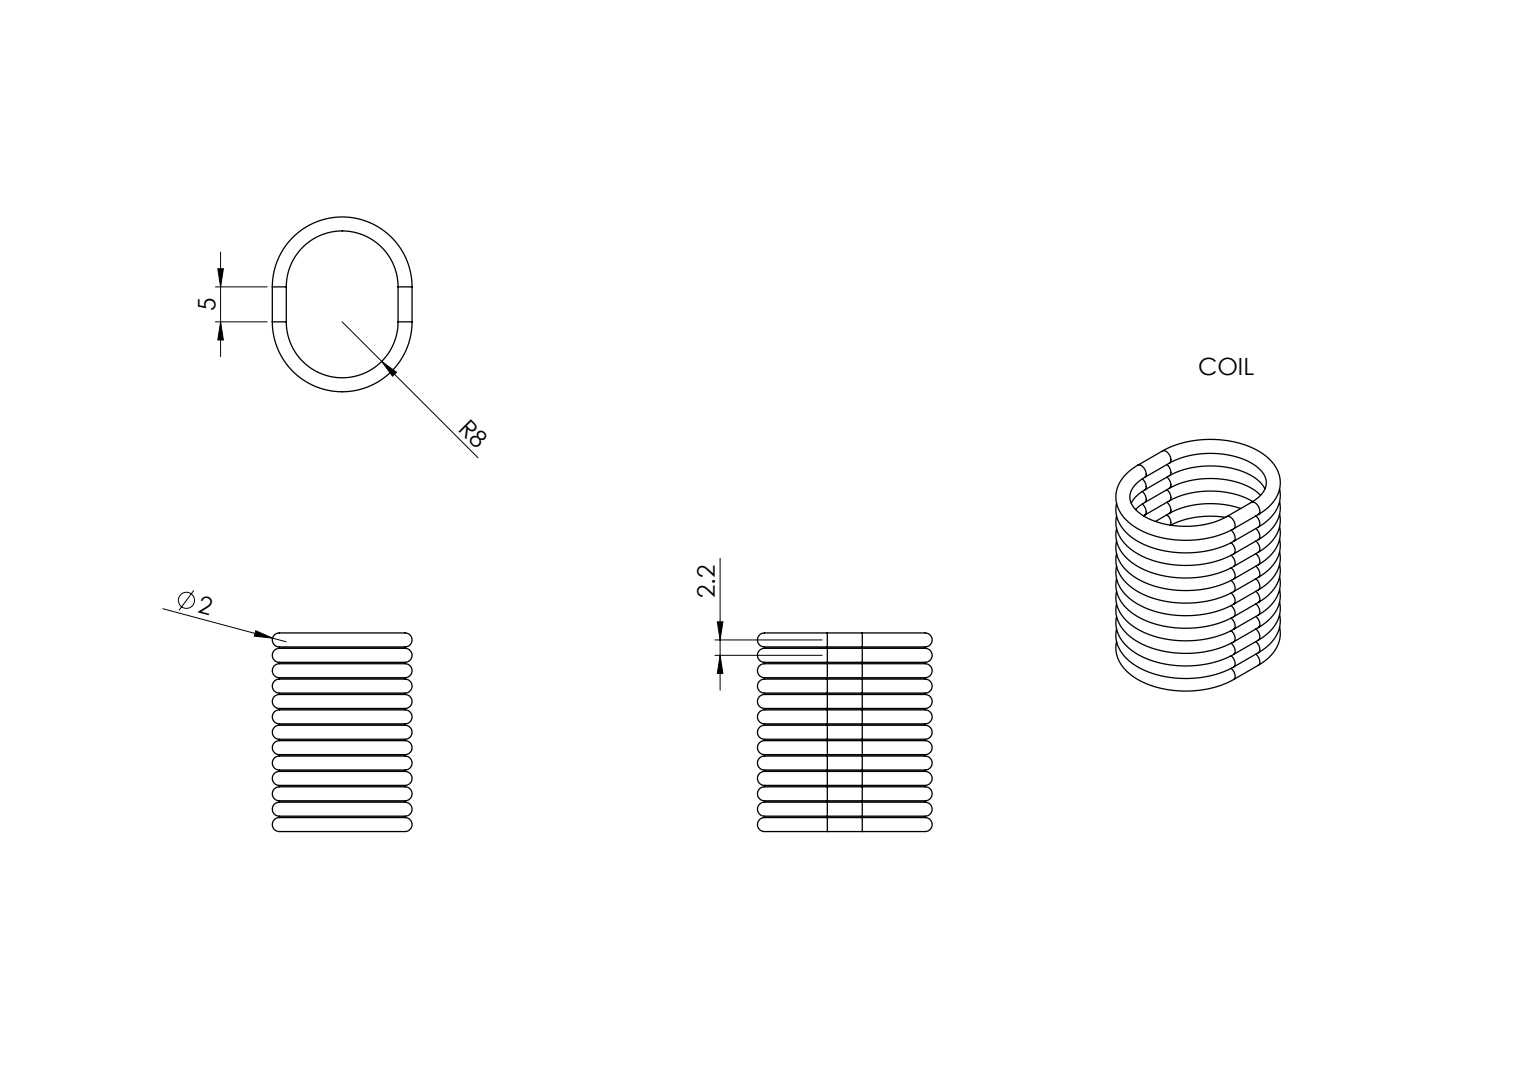
ISO-10303-21;
HEADER;
FILE_DESCRIPTION (('STEP AP214'),
    '1' );
FILE_NAME ('coil.step',
    '2026-10-25T16:39:07',
    ( '' ),
    ( '' ),
    'SwSTEP 2.0',
    'SolidWorks 2026',
    '' );
FILE_SCHEMA (( 'AUTOMOTIVE_DESIGN' ));
ENDSEC;

DATA;
#16=FACE_OUTER_BOUND ( 'NONE', #9142, .T. ) ;
#25=DIRECTION ( 'NONE',  ( 0.000000000000000000, 0.000000000000000000, -1.000000000000000000 ) ) ;
#28=CIRCLE ( 'NONE', #5350, 0.9999999999999991118 ) ;
#29=CARTESIAN_POINT ( 'NONE',  ( 10.00000000000000355, 23.19999999999999574, 2.499999999999996891 ) ) ;
#31=EDGE_CURVE ( 'NONE', #634, #10845, #10430, .T. ) ;
#33=ADVANCED_FACE ( 'NONE', ( #17875 ), #13949, .T. ) ;
#34=DIRECTION ( 'NONE',  ( -0.000000000000000000, -1.000000000000000000, -0.000000000000000000 ) ) ;
#48=DIRECTION ( 'NONE',  ( 0.000000000000000000, 0.000000000000000000, -1.000000000000000000 ) ) ;
#51=DIRECTION ( 'NONE',  ( 1.000000000000000000, 0.000000000000000000, -4.336808689942021680E-16 ) ) ;
#56=DIRECTION ( 'NONE',  ( -3.373073425510457965E-16, 0.000000000000000000, -1.000000000000000000 ) ) ;
#59=EDGE_LOOP ( 'NONE', ( #6650, #2880, #2585, #4940 ) ) ;
#60=DIRECTION ( 'NONE',  ( -1.000000000000000000, 0.000000000000000000, 4.336808689942021680E-16 ) ) ;
#71=DIRECTION ( 'NONE',  ( 1.000000000000000000, 0.000000000000000000, 0.000000000000000000 ) ) ;
#77=CARTESIAN_POINT ( 'NONE',  ( 10.00000000000000000, 34.19999999999999574, -2.500000000000003109 ) ) ;
#80=ORIENTED_EDGE ( 'NONE', *, *, #14785, .F. ) ;
#85=EDGE_CURVE ( 'NONE', #1006, #3919, #10004, .T. ) ;
#100=AXIS2_PLACEMENT_3D ( 'NONE', #14724, #10710, #2117 ) ;
#107=CARTESIAN_POINT ( 'NONE',  ( 0.000000000000000000, 29.79999999999999716, 2.500000000000000000 ) ) ;
#108=CYLINDRICAL_SURFACE ( 'NONE', #4806, 0.9999999999999991118 ) ;
#109=( LENGTH_UNIT ( ) NAMED_UNIT ( * ) SI_UNIT ( .MILLI., .METRE. ) );
#124=( NAMED_UNIT ( * ) SI_UNIT ( $, .STERADIAN. ) SOLID_ANGLE_UNIT ( ) );
#131=EDGE_CURVE ( 'NONE', #9627, #9963, #4373, .T. ) ;
#132=ORIENTED_EDGE ( 'NONE', *, *, #13174, .F. ) ;
#136=ADVANCED_FACE ( 'NONE', ( #2566 ), #16663, .T. ) ;
#137=EDGE_CURVE ( 'NONE', #3649, #894, #1162, .T. ) ;
#139=CARTESIAN_POINT ( 'NONE',  ( 9.000000000000005329, 36.39999999999999147, 2.499999999999997335 ) ) ;
#140=VECTOR ( 'NONE', #8743, 1000.000000000000000 ) ;
#141=EDGE_CURVE ( 'NONE', #15889, #18202, #16275, .T. ) ;
#145=LINE ( 'NONE', #7551, #15141 ) ;
#148=ORIENTED_EDGE ( 'NONE', *, *, #10556, .T. ) ;
#153=DIRECTION ( 'NONE',  ( 0.000000000000000000, 0.000000000000000000, 1.000000000000000000 ) ) ;
#156=VERTEX_POINT ( 'NONE', #15172 ) ;
#165=LINE ( 'NONE', #4426, #8792 ) ;
#168=CARTESIAN_POINT ( 'NONE',  ( 9.000000000000001776, 20.99999999999999289, -2.500000000000002665 ) ) ;
#170=ORIENTED_EDGE ( 'NONE', *, *, #9208, .T. ) ;
#175=AXIS2_PLACEMENT_3D ( 'NONE', #15900, #11338, #4486 ) ;
#181=DIRECTION ( 'NONE',  ( 1.000000000000000000, 0.000000000000000000, 0.000000000000000000 ) ) ;
#186=CIRCLE ( 'NONE', #5222, 0.9999999999999991118 ) ;
#188=DIRECTION ( 'NONE',  ( -0.000000000000000000, -1.000000000000000000, -0.000000000000000000 ) ) ;
#189=ORIENTED_EDGE ( 'NONE', *, *, #16096, .T. ) ;
#193=DIRECTION ( 'NONE',  ( 0.000000000000000000, 0.000000000000000000, -1.000000000000000000 ) ) ;
#213=DIRECTION ( 'NONE',  ( 1.000000000000000000, 0.000000000000000000, 0.000000000000000000 ) ) ;
#225=ADVANCED_FACE ( 'NONE', ( #14226 ), #13254, .T. ) ;
#226=CLOSED_SHELL ( 'NONE', ( #8070, #9759, #11243, #8369, #10714, #5967, #5501, #385, #7224, #136 ) ) ;
#231=AXIS2_PLACEMENT_3D ( 'NONE', #14903, #8098, #17958 ) ;
#232=CARTESIAN_POINT ( 'NONE',  ( 9.000000000000005329, 23.19999999999999574, 2.499999999999997335 ) ) ;
#238=EDGE_CURVE ( 'NONE', #14275, #456, #5568, .T. ) ;
#253=ORIENTED_EDGE ( 'NONE', *, *, #12378, .T. ) ;
#255=TOROIDAL_SURFACE ( 'NONE', #10616, 9.000000000000001776, 0.9999999999999991118 ) ;
#262=ORIENTED_EDGE ( 'NONE', *, *, #17903, .F. ) ;
#266=DIRECTION ( 'NONE',  ( -0.000000000000000000, -1.000000000000000000, -0.000000000000000000 ) ) ;
#268=EDGE_LOOP ( 'NONE', ( #17033, #4613, #7602, #12216 ) ) ;
#276=AXIS2_PLACEMENT_3D ( 'NONE', #2238, #8890, #9173 ) ;
#286=CIRCLE ( 'NONE', #5316, 8.000000000000001776 ) ;
#290=DIRECTION ( 'NONE',  ( 0.000000000000000000, 0.000000000000000000, 1.000000000000000000 ) ) ;
#294=FACE_OUTER_BOUND ( 'NONE', #4878, .T. ) ;
#296=CARTESIAN_POINT ( 'NONE',  ( -1.734723475976807094E-15, 38.59999999999999432, -2.500000000000000000 ) ) ;
#304=CARTESIAN_POINT ( 'NONE',  ( 8.000000000000001776, 16.59999999999999787, -2.500000000000002220 ) ) ;
#311=DIRECTION ( 'NONE',  ( 1.000000000000000000, 0.000000000000000000, -4.336808689942021680E-16 ) ) ;
#314=EDGE_CURVE ( 'NONE', #17692, #15689, #18053, .T. ) ;
#325=ORIENTED_EDGE ( 'NONE', *, *, #7933, .F. ) ;
#327=CIRCLE ( 'NONE', #8019, 0.9999999999999991118 ) ;
#335=DIRECTION ( 'NONE',  ( 0.000000000000000000, 0.000000000000000000, 1.000000000000000000 ) ) ;
#338=CARTESIAN_POINT ( 'NONE',  ( -8.000000000000003553, 20.99999999999999289, -2.500000000000001776 ) ) ;
#343=EDGE_LOOP ( 'NONE', ( #3432, #4004, #414, #10263 ) ) ;
#345=DIRECTION ( 'NONE',  ( 1.000000000000000000, 0.000000000000000000, 0.000000000000000000 ) ) ;
#347=DIRECTION ( 'NONE',  ( 0.000000000000000000, 0.000000000000000000, -1.000000000000000000 ) ) ;
#363=ORIENTED_EDGE ( 'NONE', *, *, #10501, .T. ) ;
#375=EDGE_CURVE ( 'NONE', #12413, #5462, #9445, .T. ) ;
#377=DIRECTION ( 'NONE',  ( -1.000000000000000000, 0.000000000000000000, 4.336808689942021680E-16 ) ) ;
#378=CIRCLE ( 'NONE', #5105, 0.9999999999999991118 ) ;
#382=ADVANCED_FACE ( 'NONE', ( #6168 ), #798, .T. ) ;
#385=ADVANCED_FACE ( 'NONE', ( #4681 ), #10332, .T. ) ;
#406=DIRECTION ( 'NONE',  ( -0.000000000000000000, -1.000000000000000000, -0.000000000000000000 ) ) ;
#414=ORIENTED_EDGE ( 'NONE', *, *, #4650, .T. ) ;
#420=DIRECTION ( 'NONE',  ( -0.000000000000000000, -1.000000000000000000, -0.000000000000000000 ) ) ;
#426=DIRECTION ( 'NONE',  ( -0.000000000000000000, -1.000000000000000000, -0.000000000000000000 ) ) ;
#427=LINE ( 'NONE', #3021, #14208 ) ;
#429=DIRECTION ( 'NONE',  ( 0.000000000000000000, 0.000000000000000000, 1.000000000000000000 ) ) ;
#443=( LENGTH_UNIT ( ) NAMED_UNIT ( * ) SI_UNIT ( .MILLI., .METRE. ) );
#454=DIRECTION ( 'NONE',  ( 3.469446951953612217E-16, -0.000000000000000000, 1.000000000000000000 ) ) ;
#456=VERTEX_POINT ( 'NONE', #14988 ) ;
#466=ORIENTED_EDGE ( 'NONE', *, *, #14601, .T. ) ;
#467=LINE ( 'NONE', #4822, #15982 ) ;
#469=DIRECTION ( 'NONE',  ( -4.915049848600951133E-16, 0.000000000000000000, -1.000000000000000000 ) ) ;
#473=ORIENTED_EDGE ( 'NONE', *, *, #4672, .F. ) ;
#474=AXIS2_PLACEMENT_3D ( 'NONE', #12018, #10254, #3231 ) ;
#477=EDGE_CURVE ( 'NONE', #6613, #1681, #7918, .T. ) ;
#484=DIRECTION ( 'NONE',  ( 0.000000000000000000, 0.000000000000000000, -1.000000000000000000 ) ) ;
#490=AXIS2_PLACEMENT_3D ( 'NONE', #9577, #2373, #2640 ) ;
#512=ORIENTED_EDGE ( 'NONE', *, *, #13369, .F. ) ;
#520=EDGE_CURVE ( 'NONE', #156, #17729, #13398, .T. ) ;
#524=DIRECTION ( 'NONE',  ( 0.000000000000000000, 0.000000000000000000, -1.000000000000000000 ) ) ;
#533=ORIENTED_EDGE ( 'NONE', *, *, #16187, .T. ) ;
#537=( NAMED_UNIT ( * ) PLANE_ANGLE_UNIT ( ) SI_UNIT ( $, .RADIAN. ) );
#562=ORIENTED_EDGE ( 'NONE', *, *, #12720, .F. ) ;
#565=CIRCLE ( 'NONE', #15638, 8.000000000000001776 ) ;
#567=ORIENTED_EDGE ( 'NONE', *, *, #8137, .F. ) ;
#573=AXIS2_PLACEMENT_3D ( 'NONE', #13525, #13619, #11017 ) ;
#579=DIRECTION ( 'NONE',  ( -3.469446951953613696E-16, -0.000000000000000000, -1.000000000000000000 ) ) ;
#583=LINE ( 'NONE', #2071, #18170 ) ;
#591=LINE ( 'NONE', #14501, #12766 ) ;
#594=DIRECTION ( 'NONE',  ( 0.000000000000000000, 0.000000000000000000, -1.000000000000000000 ) ) ;
#601=CIRCLE ( 'NONE', #17798, 0.9999999999999991118 ) ;
#606=DIRECTION ( 'NONE',  ( 0.000000000000000000, 0.000000000000000000, -1.000000000000000000 ) ) ;
#608=AXIS2_PLACEMENT_3D ( 'NONE', #7534, #13468, #14602 ) ;
#614=FACE_OUTER_BOUND ( 'NONE', #3164, .T. ) ;
#616=CARTESIAN_POINT ( 'NONE',  ( -1.734723475976807094E-15, 31.99999999999999289, -2.500000000000000000 ) ) ;
#628=LINE ( 'NONE', #9232, #14321 ) ;
#630=APPLICATION_CONTEXT ( 'automotive_design' ) ;
#634=VERTEX_POINT ( 'NONE', #16468 ) ;
#644=DIRECTION ( 'NONE',  ( -4.915049848600951133E-16, 0.000000000000000000, -1.000000000000000000 ) ) ;
#648=CARTESIAN_POINT ( 'NONE',  ( 10.00000000000000355, 27.59999999999999432, 2.499999999999996891 ) ) ;
#654=AXIS2_PLACEMENT_3D ( 'NONE', #4844, #10493, #1896 ) ;
#669=DIRECTION ( 'NONE',  ( -1.000000000000000000, 0.000000000000000000, 4.336808689942021680E-16 ) ) ;
#676=AXIS2_PLACEMENT_3D ( 'NONE', #7188, #2849, #8663 ) ;
#678=MECHANICAL_DESIGN_GEOMETRIC_PRESENTATION_REPRESENTATION('',(#17571),#3617);
#685=CYLINDRICAL_SURFACE ( 'NONE', #4943, 0.9999999999999991118 ) ;
#686=AXIS2_PLACEMENT_3D ( 'NONE', #9405, #9497, #896 ) ;
#688=( GEOMETRIC_REPRESENTATION_CONTEXT ( 3 ) GLOBAL_UNCERTAINTY_ASSIGNED_CONTEXT ( ( #16960 ) ) GLOBAL_UNIT_ASSIGNED_CONTEXT ( ( #13427, #13926, #10357 ) ) REPRESENTATION_CONTEXT ( 'NONE', 'WORKASPACE' ) );
#694=LINE ( 'NONE', #11983, #5859 ) ;
#709=AXIS2_PLACEMENT_3D ( 'NONE', #11637, #13032, #6365 ) ;
#719=ORIENTED_EDGE ( 'NONE', *, *, #15424, .F. ) ;
#721=ADVANCED_FACE ( 'NONE', ( #15892 ), #7066, .T. ) ;
#723=VERTEX_POINT ( 'NONE', #9855 ) ;
#729=DIRECTION ( 'NONE',  ( 0.000000000000000000, 0.000000000000000000, -1.000000000000000000 ) ) ;
#730=DIRECTION ( 'NONE',  ( -0.000000000000000000, -1.000000000000000000, -0.000000000000000000 ) ) ;
#735=ORIENTED_EDGE ( 'NONE', *, *, #4911, .T. ) ;
#738=ORIENTED_EDGE ( 'NONE', *, *, #3822, .F. ) ;
#739=ORIENTED_EDGE ( 'NONE', *, *, #2645, .F. ) ;
#742=( NAMED_UNIT ( * ) PLANE_ANGLE_UNIT ( ) SI_UNIT ( $, .RADIAN. ) );
#746=ORIENTED_EDGE ( 'NONE', *, *, #4495, .T. ) ;
#764=DIRECTION ( 'NONE',  ( 1.000000000000000000, 0.000000000000000000, 0.000000000000000000 ) ) ;
#772=CARTESIAN_POINT ( 'NONE',  ( 9.000000000000000000, 34.19999999999999574, -2.500000000000001332 ) ) ;
#776=ORIENTED_EDGE ( 'NONE', *, *, #13288, .T. ) ;
#785=DIRECTION ( 'NONE',  ( 1.000000000000000000, 0.000000000000000000, -4.336808689942021680E-16 ) ) ;
#790=AXIS2_PLACEMENT_3D ( 'NONE', #12105, #17977, #16580 ) ;
#793=CYLINDRICAL_SURFACE ( 'NONE', #838, 0.9999999999999991118 ) ;
#798=CYLINDRICAL_SURFACE ( 'NONE', #13600, 0.9999999999999991118 ) ;
#802=EDGE_CURVE ( 'NONE', #17357, #10052, #5688, .T. ) ;
#809=CIRCLE ( 'NONE', #6115, 10.00000000000000000 ) ;
#812=DIRECTION ( 'NONE',  ( -1.000000000000000000, 0.000000000000000000, 4.336808689942021680E-16 ) ) ;
#820=LINE ( 'NONE', #12114, #10678 ) ;
#827=CARTESIAN_POINT ( 'NONE',  ( 9.000000000000000000, 18.79999999999999361, -2.500000000000001332 ) ) ;
#828=( NAMED_UNIT ( * ) PLANE_ANGLE_UNIT ( ) SI_UNIT ( $, .RADIAN. ) );
#832=EDGE_LOOP ( 'NONE', ( #12160, #80, #2979, #5721 ) ) ;
#835=ORIENTED_EDGE ( 'NONE', *, *, #17640, .T. ) ;
#837=DIRECTION ( 'NONE',  ( -0.000000000000000000, -1.000000000000000000, -0.000000000000000000 ) ) ;
#838=AXIS2_PLACEMENT_3D ( 'NONE', #6440, #13568, #4956 ) ;
#844=EDGE_CURVE ( 'NONE', #3667, #1028, #3554, .T. ) ;
#862=CIRCLE ( 'NONE', #17761, 0.9999999999999991118 ) ;
#863=DIRECTION ( 'NONE',  ( 0.000000000000000000, 0.000000000000000000, -1.000000000000000000 ) ) ;
#864=DIRECTION ( 'NONE',  ( 0.000000000000000000, 0.000000000000000000, -1.000000000000000000 ) ) ;
#867=EDGE_LOOP ( 'NONE', ( #3646, #10246, #14638, #9895 ) ) ;
#870=EDGE_CURVE ( 'NONE', #10092, #12622, #898, .T. ) ;
#871=DIRECTION ( 'NONE',  ( 3.469446951953612217E-16, -0.000000000000000000, 1.000000000000000000 ) ) ;
#877=TOROIDAL_SURFACE ( 'NONE', #14176, 9.000000000000003553, 0.9999999999999991118 ) ;
#882=CARTESIAN_POINT ( 'NONE',  ( -9.000000000000003553, 38.59999999999999432, -2.500000000000001776 ) ) ;
#889=ORIENTED_EDGE ( 'NONE', *, *, #5357, .T. ) ;
#891=DIRECTION ( 'NONE',  ( -0.000000000000000000, -1.000000000000000000, -0.000000000000000000 ) ) ;
#894=VERTEX_POINT ( 'NONE', #16173 ) ;
#896=DIRECTION ( 'NONE',  ( 1.000000000000000000, 0.000000000000000000, -4.336808689942021680E-16 ) ) ;
#898=CIRCLE ( 'NONE', #3267, 0.9999999999999991118 ) ;
#904=VERTEX_POINT ( 'NONE', #11982 ) ;
#905=DIRECTION ( 'NONE',  ( 1.000000000000000000, 0.000000000000000000, 0.000000000000000000 ) ) ;
#907=CARTESIAN_POINT ( 'NONE',  ( -9.000000000000001776, 40.79999999999999716, 2.499999999999998224 ) ) ;
#908=CARTESIAN_POINT ( 'NONE',  ( 9.000000000000005329, 23.19999999999999574, 2.499999999999997335 ) ) ;
#910=DIRECTION ( 'NONE',  ( -0.000000000000000000, -1.000000000000000000, -0.000000000000000000 ) ) ;
#912=ORIENTED_EDGE ( 'NONE', *, *, #6249, .F. ) ;
#923=EDGE_LOOP ( 'NONE', ( #2456, #2472, #11386, #4432 ) ) ;
#940=ORIENTED_EDGE ( 'NONE', *, *, #5873, .T. ) ;
#942=DIRECTION ( 'NONE',  ( 3.469446951953612217E-16, -0.000000000000000000, 1.000000000000000000 ) ) ;
#945=ADVANCED_FACE ( 'NONE', ( #10409 ), #3647, .T. ) ;
#957=ADVANCED_FACE ( 'NONE', ( #13377 ), #17676, .T. ) ;
#960=DIRECTION ( 'NONE',  ( -1.000000000000000000, 0.000000000000000000, 4.336808689942021680E-16 ) ) ;
#969=AXIS2_PLACEMENT_3D ( 'NONE', #3169, #14578, #16244 ) ;
#976=FACE_OUTER_BOUND ( 'NONE', #6780, .T. ) ;
#978=MECHANICAL_DESIGN_GEOMETRIC_PRESENTATION_REPRESENTATION('',(#16081),#688);
#981=CARTESIAN_POINT ( 'NONE',  ( -1.734723475976807094E-15, 40.79999999999999716, -2.500000000000000000 ) ) ;
#982=DIRECTION ( 'NONE',  ( 3.469446951953612217E-16, -0.000000000000000000, 1.000000000000000000 ) ) ;
#990=CYLINDRICAL_SURFACE ( 'NONE', #8370, 0.9999999999999991118 ) ;
#993=AXIS2_PLACEMENT_3D ( 'NONE', #11771, #1974, #13258 ) ;
#1004=CARTESIAN_POINT ( 'NONE',  ( -1.734723475976807094E-15, 27.59999999999999432, -12.50000000000000000 ) ) ;
#1006=VERTEX_POINT ( 'NONE', #6050 ) ;
#1010=ORIENTED_EDGE ( 'NONE', *, *, #1403, .F. ) ;
#1017=ORIENTED_EDGE ( 'NONE', *, *, #16720, .F. ) ;
#1028=VERTEX_POINT ( 'NONE', #11795 ) ;
#1031=( NAMED_UNIT ( * ) SI_UNIT ( $, .STERADIAN. ) SOLID_ANGLE_UNIT ( ) );
#1038=UNCERTAINTY_MEASURE_WITH_UNIT (LENGTH_MEASURE( 1.000000000000000082E-05 ), #1383, 'distance_accuracy_value', 'NONE');
#1050=ADVANCED_FACE ( 'NONE', ( #6785 ), #12440, .T. ) ;
#1053=ORIENTED_EDGE ( 'NONE', *, *, #3090, .F. ) ;
#1055=CARTESIAN_POINT ( 'NONE',  ( -1.734723475976807094E-15, 40.79999999999999716, -11.50000000000000178 ) ) ;
#1086=EDGE_LOOP ( 'NONE', ( #5094, #15217, #16916, #17972 ) ) ;
#1088=AXIS2_PLACEMENT_3D ( 'NONE', #8564, #7176, #1540 ) ;
#1104=EDGE_LOOP ( 'NONE', ( #16203, #4829, #9327, #10957 ) ) ;
#1108=VERTEX_POINT ( 'NONE', #15332 ) ;
#1112=DIRECTION ( 'NONE',  ( -0.000000000000000000, -1.000000000000000000, -0.000000000000000000 ) ) ;
#1115=AXIS2_PLACEMENT_3D ( 'NONE', #2304, #910, #3862 ) ;
#1119=EDGE_CURVE ( 'NONE', #2412, #4161, #3603, .T. ) ;
#1136=CYLINDRICAL_SURFACE ( 'NONE', #6580, 0.9999999999999991118 ) ;
#1141=DIRECTION ( 'NONE',  ( -0.000000000000000000, -1.000000000000000000, -0.000000000000000000 ) ) ;
#1143=VERTEX_POINT ( 'NONE', #9381 ) ;
#1147=EDGE_LOOP ( 'NONE', ( #4251, #12196, #15311, #16287 ) ) ;
#1156=AXIS2_PLACEMENT_3D ( 'NONE', #15509, #1141, #12527 ) ;
#1157=ADVANCED_FACE ( 'NONE', ( #13647 ), #7441, .T. ) ;
#1160=AXIS2_PLACEMENT_3D ( 'NONE', #10521, #10428, #524 ) ;
#1162=CIRCLE ( 'NONE', #7024, 0.9999999999999991118 ) ;
#1165=CARTESIAN_POINT ( 'NONE',  ( -9.000000000000001776, 25.39999999999999503, 2.499999999999995559 ) ) ;
#1168=CIRCLE ( 'NONE', #3535, 8.000000000000001776 ) ;
#1173=EDGE_LOOP ( 'NONE', ( #8409, #3595, #9292, #14919 ) ) ;
#1178=EDGE_CURVE ( 'NONE', #11085, #1278, #1255, .T. ) ;
#1179=VECTOR ( 'NONE', #2036, 1000.000000000000000 ) ;
#1181=AXIS2_PLACEMENT_3D ( 'NONE', #3701, #16508, #18001 ) ;
#1184=EDGE_CURVE ( 'NONE', #13534, #6366, #11299, .T. ) ;
#1192=ORIENTED_EDGE ( 'NONE', *, *, #5126, .F. ) ;
#1200=VERTEX_POINT ( 'NONE', #14383 ) ;
#1204=VERTEX_POINT ( 'NONE', #11399 ) ;
#1207=FACE_OUTER_BOUND ( 'NONE', #13649, .T. ) ;
#1209=DIRECTION ( 'NONE',  ( 0.000000000000000000, 0.000000000000000000, 1.000000000000000000 ) ) ;
#1213=ORIENTED_EDGE ( 'NONE', *, *, #4950, .F. ) ;
#1222=CIRCLE ( 'NONE', #15714, 0.9999999999999991118 ) ;
#1234=DIRECTION ( 'NONE',  ( 0.000000000000000000, 0.000000000000000000, -1.000000000000000000 ) ) ;
#1235=FACE_OUTER_BOUND ( 'NONE', #14347, .T. ) ;
#1239=CYLINDRICAL_SURFACE ( 'NONE', #8162, 0.9999999999999991118 ) ;
#1242=ORIENTED_EDGE ( 'NONE', *, *, #9556, .F. ) ;
#1248=CARTESIAN_POINT ( 'NONE',  ( -9.000000000000001776, 16.59999999999999787, 2.499999999999998224 ) ) ;
#1255=CIRCLE ( 'NONE', #17252, 10.00000000000000000 ) ;
#1256=DIRECTION ( 'NONE',  ( -0.000000000000000000, -1.000000000000000000, -0.000000000000000000 ) ) ;
#1267=AXIS2_PLACEMENT_3D ( 'NONE', #4412, #17046, #60 ) ;
#1270=VECTOR ( 'NONE', #10266, 1000.000000000000000 ) ;
#1274=DIRECTION ( 'NONE',  ( 1.000000000000000000, 0.000000000000000000, 0.000000000000000000 ) ) ;
#1278=VERTEX_POINT ( 'NONE', #1504 ) ;
#1280=AXIS2_PLACEMENT_3D ( 'NONE', #15290, #5359, #5171 ) ;
#1282=AXIS2_PLACEMENT_3D ( 'NONE', #15593, #15687, #7048 ) ;
#1287=ADVANCED_FACE ( 'NONE', ( #14019 ), #108, .T. ) ;
#1293=EDGE_CURVE ( 'NONE', #3136, #11085, #11903, .T. ) ;
#1303=LINE ( 'NONE', #15304, #6138 ) ;
#1325=CARTESIAN_POINT ( 'NONE',  ( 0.000000000000000000, 43.00000000000000000, 2.500000000000000000 ) ) ;
#1327=ORIENTED_EDGE ( 'NONE', *, *, #4949, .T. ) ;
#1352=DIRECTION ( 'NONE',  ( 1.000000000000000000, 0.000000000000000000, 0.000000000000000000 ) ) ;
#1353=ORIENTED_EDGE ( 'NONE', *, *, #13621, .F. ) ;
#1359=FACE_OUTER_BOUND ( 'NONE', #10839, .T. ) ;
#1365=CARTESIAN_POINT ( 'NONE',  ( 9.000000000000000000, 16.59999999999999787, -2.500000000000001332 ) ) ;
#1368=ORIENTED_EDGE ( 'NONE', *, *, #5357, .F. ) ;
#1369=DIRECTION ( 'NONE',  ( -0.000000000000000000, -1.000000000000000000, -0.000000000000000000 ) ) ;
#1372=UNCERTAINTY_MEASURE_WITH_UNIT (LENGTH_MEASURE( 1.000000000000000082E-05 ), #11257, 'distance_accuracy_value', 'NONE');
#1380=ORIENTED_EDGE ( 'NONE', *, *, #7959, .T. ) ;
#1383=( LENGTH_UNIT ( ) NAMED_UNIT ( * ) SI_UNIT ( .MILLI., .METRE. ) );
#1389=CARTESIAN_POINT ( 'NONE',  ( -9.000000000000003553, 23.19999999999999574, -2.500000000000001776 ) ) ;
#1403=EDGE_CURVE ( 'NONE', #2406, #9649, #16961, .T. ) ;
#1407=AXIS2_PLACEMENT_3D ( 'NONE', #15441, #6800, #12543 ) ;
#1413=CYLINDRICAL_SURFACE ( 'NONE', #6750, 0.9999999999999991118 ) ;
#1418=DIRECTION ( 'NONE',  ( 3.469446951953612217E-16, -0.000000000000000000, 1.000000000000000000 ) ) ;
#1425=CIRCLE ( 'NONE', #11163, 0.9999999999999991118 ) ;
#1430=DIRECTION ( 'NONE',  ( -0.000000000000000000, -1.000000000000000000, -0.000000000000000000 ) ) ;
#1432=CIRCLE ( 'NONE', #11778, 0.9999999999999991118 ) ;
#1436=FACE_OUTER_BOUND ( 'NONE', #16735, .T. ) ;
#1439=ORIENTED_EDGE ( 'NONE', *, *, #1986, .T. ) ;
#1450=CARTESIAN_POINT ( 'NONE',  ( -1.734723475976807094E-15, 36.39999999999999147, -2.500000000000000000 ) ) ;
#1452=FACE_OUTER_BOUND ( 'NONE', #3465, .T. ) ;
#1453=EDGE_CURVE ( 'NONE', #14652, #12298, #10116, .T. ) ;
#1455=LINE ( 'NONE', #2670, #12411 ) ;
#1464=AXIS2_PLACEMENT_3D ( 'NONE', #17122, #15459, #11528 ) ;
#1470=CIRCLE ( 'NONE', #5021, 0.9999999999999991118 ) ;
#1473=ADVANCED_FACE ( 'NONE', ( #1882 ), #9003, .T. ) ;
#1478=LINE ( 'NONE', #2958, #7925 ) ;
#1481=DIRECTION ( 'NONE',  ( -4.915049848600951133E-16, 0.000000000000000000, -1.000000000000000000 ) ) ;
#1491=CIRCLE ( 'NONE', #5911, 0.9999999999999991118 ) ;
#1498=DIRECTION ( 'NONE',  ( 1.000000000000000000, 0.000000000000000000, -4.336808689942021680E-16 ) ) ;
#1499=EDGE_LOOP ( 'NONE', ( #16781, #12095, #7487, #14745 ) ) ;
#1504=CARTESIAN_POINT ( 'NONE',  ( 9.999999999999998224, 27.59999999999999432, -2.500000000000001776 ) ) ;
#1506=ORIENTED_EDGE ( 'NONE', *, *, #18083, .T. ) ;
#1512=EDGE_CURVE ( 'NONE', #5839, #5725, #15475, .T. ) ;
#1518=CIRCLE ( 'NONE', #1814, 0.9999999999999991118 ) ;
#1522=CARTESIAN_POINT ( 'NONE',  ( -1.734723475976807094E-15, 31.99999999999999289, -11.50000000000000178 ) ) ;
#1526=FACE_OUTER_BOUND ( 'NONE', #6394, .T. ) ;
#1531=AXIS2_PLACEMENT_3D ( 'NONE', #4749, #17198, #10301 ) ;
#1532=FACE_OUTER_BOUND ( 'NONE', #7483, .T. ) ;
#1540=DIRECTION ( 'NONE',  ( 0.000000000000000000, 0.000000000000000000, -1.000000000000000000 ) ) ;
#1553=MANIFOLD_SOLID_BREP ( 'LPattern6[5]', #11416 ) ;
#1554=ORIENTED_EDGE ( 'NONE', *, *, #5294, .F. ) ;
#1559=( NAMED_UNIT ( * ) SI_UNIT ( $, .STERADIAN. ) SOLID_ANGLE_UNIT ( ) );
#1560=DIRECTION ( 'NONE',  ( 0.000000000000000000, 0.000000000000000000, -1.000000000000000000 ) ) ;
#1561=CARTESIAN_POINT ( 'NONE',  ( 9.000000000000000000, 29.79999999999999716, -2.500000000000001332 ) ) ;
#1565=CARTESIAN_POINT ( 'NONE',  ( -8.000000000000003553, 38.59999999999999432, -2.500000000000001776 ) ) ;
#1567=VERTEX_POINT ( 'NONE', #15310 ) ;
#1569=FACE_OUTER_BOUND ( 'NONE', #11023, .T. ) ;
#1578=AXIS2_PLACEMENT_3D ( 'NONE', #14959, #10574, #16159 ) ;
#1579=VERTEX_POINT ( 'NONE', #5191 ) ;
#1581=CIRCLE ( 'NONE', #11934, 0.9999999999999991118 ) ;
#1583=ORIENTED_EDGE ( 'NONE', *, *, #1403, .T. ) ;
#1590=VECTOR ( 'NONE', #3105, 1000.000000000000000 ) ;
#1592=ORIENTED_EDGE ( 'NONE', *, *, #16531, .F. ) ;
#1595=( NAMED_UNIT ( * ) PLANE_ANGLE_UNIT ( ) SI_UNIT ( $, .RADIAN. ) );
#1610=DIRECTION ( 'NONE',  ( -1.000000000000000000, 0.000000000000000000, 0.000000000000000000 ) ) ;
#1619=LINE ( 'NONE', #15536, #1590 ) ;
#1631=DIRECTION ( 'NONE',  ( 0.000000000000000000, 0.000000000000000000, -1.000000000000000000 ) ) ;
#1647=AXIS2_PLACEMENT_3D ( 'NONE', #18229, #12539, #25 ) ;
#1652=DIRECTION ( 'NONE',  ( 0.000000000000000000, 0.000000000000000000, -1.000000000000000000 ) ) ;
#1653=DIRECTION ( 'NONE',  ( 3.469446951953612217E-16, -0.000000000000000000, 1.000000000000000000 ) ) ;
#1658=ORIENTED_EDGE ( 'NONE', *, *, #2419, .T. ) ;
#1661=LINE ( 'NONE', #13148, #1870 ) ;
#1673=DIRECTION ( 'NONE',  ( -1.000000000000000000, 0.000000000000000000, 0.000000000000000000 ) ) ;
#1675=ADVANCED_FACE ( 'NONE', ( #8333 ), #9249, .T. ) ;
#1680=CARTESIAN_POINT ( 'NONE',  ( -9.000000000000001776, 36.39999999999999147, 2.499999999999998224 ) ) ;
#1681=VERTEX_POINT ( 'NONE', #4169 ) ;
#1686=DIRECTION ( 'NONE',  ( 0.000000000000000000, 0.000000000000000000, -1.000000000000000000 ) ) ;
#1693=CLOSED_SHELL ( 'NONE', ( #4887, #6609, #18089, #13508, #4115, #17290, #2052, #11859, #3622, #7740 ) ) ;
#1704=AXIS2_PLACEMENT_3D ( 'NONE', #1389, #18104, #3890 ) ;
#1706=TOROIDAL_SURFACE ( 'NONE', #12936, 9.000000000000001776, 0.9999999999999991118 ) ;
#1710=ORIENTED_EDGE ( 'NONE', *, *, #12163, .F. ) ;
#1713=DIRECTION ( 'NONE',  ( -3.373073425510457965E-16, 0.000000000000000000, -1.000000000000000000 ) ) ;
#1731=( GEOMETRIC_REPRESENTATION_CONTEXT ( 3 ) GLOBAL_UNCERTAINTY_ASSIGNED_CONTEXT ( ( #5628 ) ) GLOBAL_UNIT_ASSIGNED_CONTEXT ( ( #5420, #4026, #8547 ) ) REPRESENTATION_CONTEXT ( 'NONE', 'WORKASPACE' ) );
#1734=ORIENTED_EDGE ( 'NONE', *, *, #7963, .F. ) ;
#1747=EDGE_CURVE ( 'NONE', #13697, #17672, #3242, .T. ) ;
#1748=AXIS2_PLACEMENT_3D ( 'NONE', #8901, #11773, #17469 ) ;
#1750=AXIS2_PLACEMENT_3D ( 'NONE', #2805, #6779, #12435 ) ;
#1757=ORIENTED_EDGE ( 'NONE', *, *, #10319, .T. ) ;
#1760=ORIENTED_EDGE ( 'NONE', *, *, #16945, .T. ) ;
#1762=DIRECTION ( 'NONE',  ( -1.000000000000000000, 0.000000000000000000, 4.336808689942021680E-16 ) ) ;
#1763=CARTESIAN_POINT ( 'NONE',  ( -10.00000000000000000, 20.99999999999999289, 2.499999999999996003 ) ) ;
#1768=TOROIDAL_SURFACE ( 'NONE', #14807, 9.000000000000003553, 0.9999999999999991118 ) ;
#1784=CYLINDRICAL_SURFACE ( 'NONE', #13376, 0.9999999999999991118 ) ;
#1786=DIRECTION ( 'NONE',  ( -1.000000000000000000, 0.000000000000000000, 4.336808689942021680E-16 ) ) ;
#1798=DIRECTION ( 'NONE',  ( 1.000000000000000000, 0.000000000000000000, 0.000000000000000000 ) ) ;
#1799=CIRCLE ( 'NONE', #16312, 0.9999999999999991118 ) ;
#1800=LINE ( 'NONE', #11327, #7109 ) ;
#1802=ORIENTED_EDGE ( 'NONE', *, *, #4978, .T. ) ;
#1814=AXIS2_PLACEMENT_3D ( 'NONE', #5071, #6646, #10726 ) ;
#1820=DIRECTION ( 'NONE',  ( -0.000000000000000000, -1.000000000000000000, -0.000000000000000000 ) ) ;
#1825=AXIS2_PLACEMENT_3D ( 'NONE', #16288, #2288, #9039 ) ;
#1840=DIRECTION ( 'NONE',  ( 0.000000000000000000, 0.000000000000000000, 1.000000000000000000 ) ) ;
#1843=CARTESIAN_POINT ( 'NONE',  ( 0.000000000000000000, 36.39999999999999147, 2.500000000000000000 ) ) ;
#1845=EDGE_CURVE ( 'NONE', #15990, #1204, #16138, .T. ) ;
#1852=DIRECTION ( 'NONE',  ( 0.000000000000000000, 0.000000000000000000, -1.000000000000000000 ) ) ;
#1854=ORIENTED_EDGE ( 'NONE', *, *, #15457, .T. ) ;
#1857=DIRECTION ( 'NONE',  ( -1.000000000000000000, 0.000000000000000000, 4.336808689942021680E-16 ) ) ;
#1867=EDGE_LOOP ( 'NONE', ( #7751, #5084, #735, #6442 ) ) ;
#1869=CARTESIAN_POINT ( 'NONE',  ( 0.000000000000000000, 27.59999999999999432, 2.500000000000000000 ) ) ;
#1870=VECTOR ( 'NONE', #12957, 1000.000000000000000 ) ;
#1874=ADVANCED_FACE ( 'NONE', ( #11946 ), #6876, .T. ) ;
#1877=EDGE_LOOP ( 'NONE', ( #13570, #13814, #12192, #17396 ) ) ;
#1881=AXIS2_PLACEMENT_3D ( 'NONE', #14582, #10196, #18241 ) ;
#1882=FACE_OUTER_BOUND ( 'NONE', #13197, .T. ) ;
#1887=DIRECTION ( 'NONE',  ( -0.000000000000000000, -1.000000000000000000, -0.000000000000000000 ) ) ;
#1895=EDGE_CURVE ( 'NONE', #12298, #3719, #14461, .T. ) ;
#1896=DIRECTION ( 'NONE',  ( 0.000000000000000000, 0.000000000000000000, -1.000000000000000000 ) ) ;
#1897=AXIS2_PLACEMENT_3D ( 'NONE', #5629, #11272, #7371 ) ;
#1898=DIRECTION ( 'NONE',  ( 0.000000000000000000, 0.000000000000000000, -1.000000000000000000 ) ) ;
#1900=CARTESIAN_POINT ( 'NONE',  ( 9.000000000000005329, 34.19999999999999574, 2.499999999999997335 ) ) ;
#1910=AXIS2_PLACEMENT_3D ( 'NONE', #10415, #8929, #785 ) ;
#1911=PRODUCT ( 'coil', 'coil', '', ( #8018 ) ) ;
#1921=EDGE_CURVE ( 'NONE', #17611, #11426, #378, .T. ) ;
#1923=EDGE_CURVE ( 'NONE', #4547, #7574, #10132, .T. ) ;
#1924=DIRECTION ( 'NONE',  ( 0.000000000000000000, 0.000000000000000000, 1.000000000000000000 ) ) ;
#1926=DIRECTION ( 'NONE',  ( 0.000000000000000000, 0.000000000000000000, -1.000000000000000000 ) ) ;
#1932=LINE ( 'NONE', #4780, #10114 ) ;
#1941=CYLINDRICAL_SURFACE ( 'NONE', #9557, 0.9999999999999991118 ) ;
#1945=CARTESIAN_POINT ( 'NONE',  ( -1.734723475976807094E-15, 43.00000000000000000, -2.500000000000000000 ) ) ;
#1948=ORIENTED_EDGE ( 'NONE', *, *, #13369, .T. ) ;
#1953=ORIENTED_EDGE ( 'NONE', *, *, #844, .T. ) ;
#1964=CARTESIAN_POINT ( 'NONE',  ( 9.000000000000000000, 31.99999999999999289, -2.500000000000001332 ) ) ;
#1970=FACE_OUTER_BOUND ( 'NONE', #15511, .T. ) ;
#1972=TOROIDAL_SURFACE ( 'NONE', #11129, 9.000000000000001776, 0.9999999999999991118 ) ;
#1974=DIRECTION ( 'NONE',  ( -4.915049848600951133E-16, 0.000000000000000000, -1.000000000000000000 ) ) ;
#1984=EDGE_CURVE ( 'NONE', #2199, #904, #13092, .T. ) ;
#1986=EDGE_CURVE ( 'NONE', #4985, #13359, #1661, .T. ) ;
#1993=ORIENTED_EDGE ( 'NONE', *, *, #1921, .F. ) ;
#2004=MANIFOLD_SOLID_BREP ( 'LPattern6[4]', #1693 ) ;
#2014=LINE ( 'NONE', #17787, #5367 ) ;
#2021=STYLED_ITEM('',(#18396),#13775);
#2023=VECTOR ( 'NONE', #15820, 1000.000000000000000 ) ;
#2032=DIRECTION ( 'NONE',  ( 0.000000000000000000, 0.000000000000000000, -1.000000000000000000 ) ) ;
#2034=DIRECTION ( 'NONE',  ( 0.000000000000000000, 0.000000000000000000, -1.000000000000000000 ) ) ;
#2035=VECTOR ( 'NONE', #2363, 1000.000000000000000 ) ;
#2036=DIRECTION ( 'NONE',  ( 3.469446951953612217E-16, -0.000000000000000000, 1.000000000000000000 ) ) ;
#2038=ORIENTED_EDGE ( 'NONE', *, *, #9326, .F. ) ;
#2041=DIRECTION ( 'NONE',  ( 0.000000000000000000, 0.000000000000000000, 1.000000000000000000 ) ) ;
#2050=( GEOMETRIC_REPRESENTATION_CONTEXT ( 3 ) GLOBAL_UNCERTAINTY_ASSIGNED_CONTEXT ( ( #18116 ) ) GLOBAL_UNIT_ASSIGNED_CONTEXT ( ( #6927, #18002, #16878 ) ) REPRESENTATION_CONTEXT ( 'NONE', 'WORKASPACE' ) );
#2052=ADVANCED_FACE ( 'NONE', ( #14456 ), #17582, .T. ) ;
#2056=DIRECTION ( 'NONE',  ( 0.000000000000000000, 0.000000000000000000, -1.000000000000000000 ) ) ;
#2062=CIRCLE ( 'NONE', #2370, 0.9999999999999991118 ) ;
#2071=CARTESIAN_POINT ( 'NONE',  ( -10.00000000000000000, 29.79999999999999716, 2.499999999999996003 ) ) ;
#2082=DIRECTION ( 'NONE',  ( 1.000000000000000000, 0.000000000000000000, 0.000000000000000000 ) ) ;
#2084=DIRECTION ( 'NONE',  ( 1.000000000000000000, 0.000000000000000000, 0.000000000000000000 ) ) ;
#2085=ORIENTED_EDGE ( 'NONE', *, *, #15852, .F. ) ;
#2087=DIRECTION ( 'NONE',  ( -1.000000000000000000, 0.000000000000000000, 0.000000000000000000 ) ) ;
#2096=CARTESIAN_POINT ( 'NONE',  ( -1.734723475976807094E-15, 16.59999999999999787, -12.50000000000000000 ) ) ;
#2101=LINE ( 'NONE', #14709, #140 ) ;
#2106=DIRECTION ( 'NONE',  ( 0.000000000000000000, 0.000000000000000000, 1.000000000000000000 ) ) ;
#2108=ORIENTED_EDGE ( 'NONE', *, *, #10220, .T. ) ;
#2117=DIRECTION ( 'NONE',  ( 0.000000000000000000, 0.000000000000000000, -1.000000000000000000 ) ) ;
#2119=ORIENTED_EDGE ( 'NONE', *, *, #13222, .T. ) ;
#2124=FACE_OUTER_BOUND ( 'NONE', #10407, .T. ) ;
#2131=VERTEX_POINT ( 'NONE', #13143 ) ;
#2134=EDGE_LOOP ( 'NONE', ( #8973, #7928, #13787, #3984 ) ) ;
#2135=ORIENTED_EDGE ( 'NONE', *, *, #4168, .F. ) ;
#2142=MECHANICAL_DESIGN_GEOMETRIC_PRESENTATION_REPRESENTATION('',(#10995),#5379);
#2145=ORIENTED_EDGE ( 'NONE', *, *, #4551, .T. ) ;
#2158=DIRECTION ( 'NONE',  ( 0.000000000000000000, 0.000000000000000000, -1.000000000000000000 ) ) ;
#2163=DIRECTION ( 'NONE',  ( 0.000000000000000000, 0.000000000000000000, 1.000000000000000000 ) ) ;
#2166=AXIS2_PLACEMENT_3D ( 'NONE', #17159, #11467, #1762 ) ;
#2173=EDGE_CURVE ( 'NONE', #14275, #5635, #6318, .T. ) ;
#2174=CARTESIAN_POINT ( 'NONE',  ( -9.000000000000001776, 43.00000000000000000, 2.499999999999995559 ) ) ;
#2178=DIRECTION ( 'NONE',  ( 0.000000000000000000, 0.000000000000000000, 1.000000000000000000 ) ) ;
#2180=ORIENTED_EDGE ( 'NONE', *, *, #11064, .F. ) ;
#2182=DIRECTION ( 'NONE',  ( 3.469446951953612217E-16, -0.000000000000000000, 1.000000000000000000 ) ) ;
#2190=DIRECTION ( 'NONE',  ( 0.000000000000000000, 0.000000000000000000, -1.000000000000000000 ) ) ;
#2192=VECTOR ( 'NONE', #12760, 1000.000000000000000 ) ;
#2196=DIRECTION ( 'NONE',  ( -0.000000000000000000, -1.000000000000000000, -0.000000000000000000 ) ) ;
#2199=VERTEX_POINT ( 'NONE', #11491 ) ;
#2202=CARTESIAN_POINT ( 'NONE',  ( -8.000000000000001776, 36.39999999999999147, 2.499999999999995115 ) ) ;
#2209=EDGE_CURVE ( 'NONE', #18202, #5429, #7480, .T. ) ;
#2210=EDGE_CURVE ( 'NONE', #4161, #15889, #6899, .T. ) ;
#2214=ADVANCED_FACE ( 'NONE', ( #8708 ), #13710, .T. ) ;
#2219=DIRECTION ( 'NONE',  ( 0.000000000000000000, 0.000000000000000000, 1.000000000000000000 ) ) ;
#2222=AXIS2_PLACEMENT_3D ( 'NONE', #2975, #8699, #14283 ) ;
#2237=EDGE_LOOP ( 'NONE', ( #4935, #6317, #4510, #1327 ) ) ;
#2238=CARTESIAN_POINT ( 'NONE',  ( 9.000000000000000000, 20.99999999999999289, -2.500000000000001332 ) ) ;
#2247=MANIFOLD_SOLID_BREP ( 'LPattern6[12]', #16538 ) ;
#2252=ORIENTED_EDGE ( 'NONE', *, *, #8067, .T. ) ;
#2262=ADVANCED_FACE ( 'NONE', ( #10664 ), #18186, .T. ) ;
#2265=DIRECTION ( 'NONE',  ( -0.000000000000000000, -1.000000000000000000, -0.000000000000000000 ) ) ;
#2267=CARTESIAN_POINT ( 'NONE',  ( -10.00000000000000000, 29.79999999999999716, 2.499999999999998224 ) ) ;
#2276=VECTOR ( 'NONE', #5678, 1000.000000000000000 ) ;
#2288=DIRECTION ( 'NONE',  ( -0.000000000000000000, -1.000000000000000000, -0.000000000000000000 ) ) ;
#2304=CARTESIAN_POINT ( 'NONE',  ( 0.000000000000000000, 18.79999999999999361, 2.500000000000000000 ) ) ;
#2316=DIRECTION ( 'NONE',  ( 0.000000000000000000, 0.000000000000000000, -1.000000000000000000 ) ) ;
#2325=ORIENTED_EDGE ( 'NONE', *, *, #16764, .T. ) ;
#2329=CARTESIAN_POINT ( 'NONE',  ( -9.000000000000001776, 31.99999999999999289, 2.499999999999998224 ) ) ;
#2330=ADVANCED_FACE ( 'NONE', ( #10287 ), #16988, .T. ) ;
#2334=PRODUCT_DEFINITION ( 'UNKNOWN', '', #8054, #8397 ) ;
#2336=EDGE_LOOP ( 'NONE', ( #2937, #8500, #14384, #14550 ) ) ;
#2345=DIRECTION ( 'NONE',  ( -1.000000000000000000, 0.000000000000000000, 4.336808689942021680E-16 ) ) ;
#2355=VECTOR ( 'NONE', #13808, 1000.000000000000000 ) ;
#2356=DIRECTION ( 'NONE',  ( -3.373073425510457965E-16, 0.000000000000000000, -1.000000000000000000 ) ) ;
#2358=CARTESIAN_POINT ( 'NONE',  ( -9.000000000000001776, 16.59999999999999787, 2.499999999999995559 ) ) ;
#2359=ORIENTED_EDGE ( 'NONE', *, *, #16187, .F. ) ;
#2360=ORIENTED_EDGE ( 'NONE', *, *, #12355, .F. ) ;
#2362=CARTESIAN_POINT ( 'NONE',  ( -9.000000000000003553, 23.19999999999999574, -2.500000000000001776 ) ) ;
#2363=DIRECTION ( 'NONE',  ( 3.469446951953612217E-16, -0.000000000000000000, 1.000000000000000000 ) ) ;
#2370=AXIS2_PLACEMENT_3D ( 'NONE', #16701, #4061, #13897 ) ;
#2371=CARTESIAN_POINT ( 'NONE',  ( 9.000000000000001776, 18.79999999999999361, -2.500000000000002665 ) ) ;
#2372=CIRCLE ( 'NONE', #13591, 8.000000000000003553 ) ;
#2373=DIRECTION ( 'NONE',  ( -0.000000000000000000, -1.000000000000000000, -0.000000000000000000 ) ) ;
#2377=CARTESIAN_POINT ( 'NONE',  ( -1.734723475976807094E-15, 27.59999999999999432, -11.50000000000000178 ) ) ;
#2386=FACE_OUTER_BOUND ( 'NONE', #1173, .T. ) ;
#2391=AXIS2_PLACEMENT_3D ( 'NONE', #5326, #8372, #11242 ) ;
#2398=CARTESIAN_POINT ( 'NONE',  ( -1.734723475976807094E-15, 38.59999999999999432, -11.50000000000000178 ) ) ;
#2400=EDGE_LOOP ( 'NONE', ( #262, #11099, #10817, #12696 ) ) ;
#2406=VERTEX_POINT ( 'NONE', #6313 ) ;
#2410=DIRECTION ( 'NONE',  ( 3.469446951953612217E-16, -0.000000000000000000, 1.000000000000000000 ) ) ;
#2412=VERTEX_POINT ( 'NONE', #10569 ) ;
#2415=ORIENTED_EDGE ( 'NONE', *, *, #14835, .F. ) ;
#2416=EDGE_CURVE ( 'NONE', #904, #2199, #14614, .T. ) ;
#2419=EDGE_CURVE ( 'NONE', #3719, #17692, #11325, .T. ) ;
#2432=TOROIDAL_SURFACE ( 'NONE', #5066, 9.000000000000001776, 0.9999999999999991118 ) ;
#2439=VERTEX_POINT ( 'NONE', #16430 ) ;
#2443=DIRECTION ( 'NONE',  ( -1.000000000000000000, 0.000000000000000000, 4.336808689942021680E-16 ) ) ;
#2444=COLOUR_RGB ( '',0.8941176470588234615, 0.8941176470588234615, 0.8941176470588234615 ) ;
#2447=DIRECTION ( 'NONE',  ( -1.000000000000000000, 0.000000000000000000, 0.000000000000000000 ) ) ;
#2449=ORIENTED_EDGE ( 'NONE', *, *, #14993, .T. ) ;
#2450=EDGE_LOOP ( 'NONE', ( #14044, #9156, #13004, #5784 ) ) ;
#2452=DIRECTION ( 'NONE',  ( -1.000000000000000000, 0.000000000000000000, 0.000000000000000000 ) ) ;
#2456=ORIENTED_EDGE ( 'NONE', *, *, #16482, .F. ) ;
#2465=DIRECTION ( 'NONE',  ( -0.000000000000000000, -1.000000000000000000, -0.000000000000000000 ) ) ;
#2467=DIRECTION ( 'NONE',  ( -0.000000000000000000, -1.000000000000000000, -0.000000000000000000 ) ) ;
#2470=CYLINDRICAL_SURFACE ( 'NONE', #18321, 0.9999999999999991118 ) ;
#2472=ORIENTED_EDGE ( 'NONE', *, *, #6638, .T. ) ;
#2474=DIRECTION ( 'NONE',  ( 0.000000000000000000, 0.000000000000000000, -1.000000000000000000 ) ) ;
#2478=CARTESIAN_POINT ( 'NONE',  ( 10.00000000000000355, 40.79999999999999716, 2.499999999999996891 ) ) ;
#2483=EDGE_CURVE ( 'NONE', #10052, #11668, #1581, .T. ) ;
#2485=ORIENTED_EDGE ( 'NONE', *, *, #13294, .T. ) ;
#2488=ADVANCED_FACE ( 'NONE', ( #18199 ), #14307, .T. ) ;
#2490=CARTESIAN_POINT ( 'NONE',  ( 9.999999999999998224, 40.79999999999999716, -2.500000000000001776 ) ) ;
#2491=TOROIDAL_SURFACE ( 'NONE', #17297, 9.000000000000003553, 0.9999999999999991118 ) ;
#2495=CARTESIAN_POINT ( 'NONE',  ( 9.999999999999998224, 31.99999999999999289, -2.500000000000001776 ) ) ;
#2498=ORIENTED_EDGE ( 'NONE', *, *, #17032, .F. ) ;
#2502=UNCERTAINTY_MEASURE_WITH_UNIT (LENGTH_MEASURE( 1.000000000000000082E-05 ), #4384, 'distance_accuracy_value', 'NONE');
#2505=AXIS2_PLACEMENT_3D ( 'NONE', #10034, #3010, #8643 ) ;
#2513=CARTESIAN_POINT ( 'NONE',  ( -1.734723475976807094E-15, 18.79999999999999361, -2.500000000000000000 ) ) ;
#2533=TOROIDAL_SURFACE ( 'NONE', #15264, 9.000000000000001776, 0.9999999999999991118 ) ;
#2536=DIRECTION ( 'NONE',  ( -4.915049848600951133E-16, 0.000000000000000000, -1.000000000000000000 ) ) ;
#2537=DIRECTION ( 'NONE',  ( -0.000000000000000000, -1.000000000000000000, -0.000000000000000000 ) ) ;
#2561=CIRCLE ( 'NONE', #12897, 0.9999999999999991118 ) ;
#2565=CIRCLE ( 'NONE', #16784, 8.000000000000001776 ) ;
#2566=FACE_OUTER_BOUND ( 'NONE', #11461, .T. ) ;
#2575=AXIS2_PLACEMENT_3D ( 'NONE', #17037, #5790, #11166 ) ;
#2582=DIRECTION ( 'NONE',  ( -1.000000000000000000, 0.000000000000000000, 4.336808689942021680E-16 ) ) ;
#2585=ORIENTED_EDGE ( 'NONE', *, *, #4609, .T. ) ;
#2590=AXIS2_PLACEMENT_3D ( 'NONE', #17954, #2467, #8095 ) ;
#2603=ORIENTED_EDGE ( 'NONE', *, *, #802, .T. ) ;
#2627=CIRCLE ( 'NONE', #12965, 10.00000000000000178 ) ;
#2632=DIRECTION ( 'NONE',  ( -1.000000000000000000, 0.000000000000000000, 0.000000000000000000 ) ) ;
#2640=DIRECTION ( 'NONE',  ( 0.000000000000000000, 0.000000000000000000, -1.000000000000000000 ) ) ;
#2641=AXIS2_PLACEMENT_3D ( 'NONE', #13467, #2087, #11888 ) ;
#2645=EDGE_CURVE ( 'NONE', #5462, #11668, #14512, .T. ) ;
#2653=CIRCLE ( 'NONE', #13589, 0.9999999999999991118 ) ;
#2655=AXIS2_PLACEMENT_3D ( 'NONE', #4723, #837, #2056 ) ;
#2661=EDGE_CURVE ( 'NONE', #4032, #9180, #11593, .T. ) ;
#2667=MECHANICAL_DESIGN_GEOMETRIC_PRESENTATION_REPRESENTATION('',(#6507),#16887);
#2670=CARTESIAN_POINT ( 'NONE',  ( 8.000000000000001776, 36.39999999999999147, -2.500000000000002220 ) ) ;
#2680=AXIS2_PLACEMENT_3D ( 'NONE', #17603, #6529, #12085 ) ;
#2682=UNCERTAINTY_MEASURE_WITH_UNIT (LENGTH_MEASURE( 1.000000000000000082E-05 ), #8615, 'distance_accuracy_value', 'NONE');
#2685=VERTEX_POINT ( 'NONE', #5695 ) ;
#2694=AXIS2_PLACEMENT_3D ( 'NONE', #12818, #14397, #8543 ) ;
#2712=EDGE_CURVE ( 'NONE', #17357, #5462, #13674, .T. ) ;
#2726=DIRECTION ( 'NONE',  ( -1.000000000000000000, 0.000000000000000000, 4.336808689942021680E-16 ) ) ;
#2727=DIRECTION ( 'NONE',  ( -0.000000000000000000, -1.000000000000000000, -0.000000000000000000 ) ) ;
#2747=EDGE_CURVE ( 'NONE', #9609, #13697, #8343, .T. ) ;
#2751=TOROIDAL_SURFACE ( 'NONE', #9549, 9.000000000000003553, 0.9999999999999991118 ) ;
#2754=AXIS2_PLACEMENT_3D ( 'NONE', #7395, #14655, #13054 ) ;
#2756=CARTESIAN_POINT ( 'NONE',  ( -1.734723475976807094E-15, 36.39999999999999147, -12.50000000000000000 ) ) ;
#2758=DIRECTION ( 'NONE',  ( -1.000000000000000000, 0.000000000000000000, 4.336808689942021680E-16 ) ) ;
#2765=STYLED_ITEM('',(#18396),#2247);
#2782=DIRECTION ( 'NONE',  ( -3.373073425510457965E-16, 0.000000000000000000, -1.000000000000000000 ) ) ;
#2787=ORIENTED_EDGE ( 'NONE', *, *, #11924, .T. ) ;
#2789=DIRECTION ( 'NONE',  ( -1.000000000000000000, 0.000000000000000000, 4.336808689942021680E-16 ) ) ;
#2790=AXIS2_PLACEMENT_3D ( 'NONE', #1248, #15066, #16456 ) ;
#2798=EDGE_CURVE ( 'NONE', #7045, #3783, #12479, .T. ) ;
#2803=FACE_OUTER_BOUND ( 'NONE', #1086, .T. ) ;
#2805=CARTESIAN_POINT ( 'NONE',  ( -1.734723475976807094E-15, 23.19999999999999574, -2.500000000000000000 ) ) ;
#2806=VERTEX_POINT ( 'NONE', #11584 ) ;
#2807=ORIENTED_EDGE ( 'NONE', *, *, #17859, .F. ) ;
#2811=DIRECTION ( 'NONE',  ( 0.000000000000000000, 0.000000000000000000, -1.000000000000000000 ) ) ;
#2819=CARTESIAN_POINT ( 'NONE',  ( 0.000000000000000000, 16.59999999999999787, 2.500000000000000000 ) ) ;
#2820=ADVANCED_FACE ( 'NONE', ( #11490 ), #1784, .T. ) ;
#2828=EDGE_LOOP ( 'NONE', ( #9130, #7916, #14488, #9475 ) ) ;
#2838=( NAMED_UNIT ( * ) PLANE_ANGLE_UNIT ( ) SI_UNIT ( $, .RADIAN. ) );
#2842=AXIS2_PLACEMENT_3D ( 'NONE', #13415, #730, #8868 ) ;
#2845=DIRECTION ( 'NONE',  ( -1.000000000000000000, 0.000000000000000000, 4.336808689942021680E-16 ) ) ;
#2849=DIRECTION ( 'NONE',  ( -3.373073425510457965E-16, 0.000000000000000000, -1.000000000000000000 ) ) ;
#2852=ORIENTED_EDGE ( 'NONE', *, *, #10457, .F. ) ;
#2860=CARTESIAN_POINT ( 'NONE',  ( 9.000000000000000000, 25.39999999999999503, -2.500000000000001332 ) ) ;
#2861=ADVANCED_FACE ( 'NONE', ( #294 ), #11631, .T. ) ;
#2865=ADVANCED_FACE ( 'NONE', ( #5667 ), #17853, .T. ) ;
#2867=EDGE_LOOP ( 'NONE', ( #15191, #14674, #14931, #512 ) ) ;
#2868=AXIS2_PLACEMENT_3D ( 'NONE', #7528, #12901, #1898 ) ;
#2880=ORIENTED_EDGE ( 'NONE', *, *, #15246, .F. ) ;
#2890=ORIENTED_EDGE ( 'NONE', *, *, #6901, .T. ) ;
#2907=CIRCLE ( 'NONE', #3213, 10.00000000000000000 ) ;
#2908=TOROIDAL_SURFACE ( 'NONE', #3216, 9.000000000000001776, 0.9999999999999991118 ) ;
#2914=( NAMED_UNIT ( * ) PLANE_ANGLE_UNIT ( ) SI_UNIT ( $, .RADIAN. ) );
#2920=TOROIDAL_SURFACE ( 'NONE', #4376, 9.000000000000001776, 0.9999999999999991118 ) ;
#2937=ORIENTED_EDGE ( 'NONE', *, *, #17114, .F. ) ;
#2939=FACE_OUTER_BOUND ( 'NONE', #4064, .T. ) ;
#2946=CIRCLE ( 'NONE', #7375, 0.9999999999999991118 ) ;
#2948=CIRCLE ( 'NONE', #9739, 0.9999999999999991118 ) ;
#2950=CARTESIAN_POINT ( 'NONE',  ( -8.000000000000001776, 16.59999999999999787, 2.499999999999998224 ) ) ;
#2958=CARTESIAN_POINT ( 'NONE',  ( -10.00000000000000000, 25.39999999999999503, 2.499999999999996003 ) ) ;
#2959=ORIENTED_EDGE ( 'NONE', *, *, #12317, .T. ) ;
#2961=CARTESIAN_POINT ( 'NONE',  ( 9.999999999999998224, 36.39999999999999147, -2.500000000000001776 ) ) ;
#2966=EDGE_LOOP ( 'NONE', ( #739, #16320, #2603, #3520 ) ) ;
#2971=VECTOR ( 'NONE', #13182, 1000.000000000000000 ) ;
#2975=CARTESIAN_POINT ( 'NONE',  ( -9.000000000000001776, 20.99999999999999289, 2.499999999999995559 ) ) ;
#2979=ORIENTED_EDGE ( 'NONE', *, *, #7152, .T. ) ;
#2987=AXIS2_PLACEMENT_3D ( 'NONE', #15725, #429, #6167 ) ;
#2994=ADVANCED_FACE ( 'NONE', ( #5189 ), #8149, .T. ) ;
#2999=CARTESIAN_POINT ( 'NONE',  ( -9.000000000000003553, 31.99999999999999289, -2.500000000000001776 ) ) ;
#3004=ORIENTED_EDGE ( 'NONE', *, *, #8865, .F. ) ;
#3010=DIRECTION ( 'NONE',  ( -0.000000000000000000, -1.000000000000000000, -0.000000000000000000 ) ) ;
#3013=ORIENTED_EDGE ( 'NONE', *, *, #7679, .T. ) ;
#3018=CARTESIAN_POINT ( 'NONE',  ( -9.000000000000001776, 36.39999999999999147, 2.499999999999995559 ) ) ;
#3020=CARTESIAN_POINT ( 'NONE',  ( -1.734723475976807094E-15, 38.59999999999999432, -2.500000000000000000 ) ) ;
#3021=CARTESIAN_POINT ( 'NONE',  ( -10.00000000000000000, 40.79999999999999716, 2.499999999999996003 ) ) ;
#3022=DIRECTION ( 'NONE',  ( -0.000000000000000000, -1.000000000000000000, -0.000000000000000000 ) ) ;
#3030=AXIS2_PLACEMENT_3D ( 'NONE', #7456, #1481, #7394 ) ;
#3034=DIRECTION ( 'NONE',  ( 1.000000000000000000, 0.000000000000000000, 0.000000000000000000 ) ) ;
#3045=DIRECTION ( 'NONE',  ( -1.000000000000000000, 0.000000000000000000, 4.336808689942021680E-16 ) ) ;
#3050=EDGE_LOOP ( 'NONE', ( #10682, #11607, #3607, #835 ) ) ;
#3051=DIRECTION ( 'NONE',  ( -3.469446951953613696E-16, -0.000000000000000000, -1.000000000000000000 ) ) ;
#3059=ORIENTED_EDGE ( 'NONE', *, *, #5126, .T. ) ;
#3063=ORIENTED_EDGE ( 'NONE', *, *, #16478, .T. ) ;
#3064=DIRECTION ( 'NONE',  ( -0.000000000000000000, -1.000000000000000000, -0.000000000000000000 ) ) ;
#3075=DIRECTION ( 'NONE',  ( -0.000000000000000000, -1.000000000000000000, -0.000000000000000000 ) ) ;
#3087=( GEOMETRIC_REPRESENTATION_CONTEXT ( 3 ) GLOBAL_UNCERTAINTY_ASSIGNED_CONTEXT ( ( #9521 ) ) GLOBAL_UNIT_ASSIGNED_CONTEXT ( ( #13827, #5206, #8074 ) ) REPRESENTATION_CONTEXT ( 'NONE', 'WORKASPACE' ) );
#3090=EDGE_CURVE ( 'NONE', #15689, #12253, #10419, .T. ) ;
#3105=DIRECTION ( 'NONE',  ( -3.469446951953613696E-16, -0.000000000000000000, -1.000000000000000000 ) ) ;
#3107=VERTEX_POINT ( 'NONE', #5553 ) ;
#3123=DIRECTION ( 'NONE',  ( 0.000000000000000000, 0.000000000000000000, -1.000000000000000000 ) ) ;
#3134=CARTESIAN_POINT ( 'NONE',  ( -1.734723475976807094E-15, 25.39999999999999503, -2.500000000000000000 ) ) ;
#3136=VERTEX_POINT ( 'NONE', #16619 ) ;
#3138=DIRECTION ( 'NONE',  ( -3.469446951953613696E-16, -0.000000000000000000, -1.000000000000000000 ) ) ;
#3140=ORIENTED_EDGE ( 'NONE', *, *, #4221, .T. ) ;
#3150=CIRCLE ( 'NONE', #13497, 10.00000000000000178 ) ;
#3152=ORIENTED_EDGE ( 'NONE', *, *, #3822, .T. ) ;
#3160=CIRCLE ( 'NONE', #11421, 0.9999999999999991118 ) ;
#3162=CARTESIAN_POINT ( 'NONE',  ( -1.734723475976807094E-15, 43.00000000000000000, -11.50000000000000178 ) ) ;
#3164=EDGE_LOOP ( 'NONE', ( #10718, #1710, #1953, #11361 ) ) ;
#3167=DIRECTION ( 'NONE',  ( 0.000000000000000000, 0.000000000000000000, -1.000000000000000000 ) ) ;
#3169=CARTESIAN_POINT ( 'NONE',  ( 9.000000000000000000, 34.19999999999999574, -2.500000000000001332 ) ) ;
#3177=CIRCLE ( 'NONE', #3472, 0.9999999999999991118 ) ;
#3187=EDGE_LOOP ( 'NONE', ( #4711, #16801, #170, #9428 ) ) ;
#3189=CARTESIAN_POINT ( 'NONE',  ( -9.000000000000001776, 31.99999999999999289, 2.499999999999995559 ) ) ;
#3191=VERTEX_POINT ( 'NONE', #2961 ) ;
#3206=DIRECTION ( 'NONE',  ( 0.000000000000000000, 0.000000000000000000, -1.000000000000000000 ) ) ;
#3207=ADVANCED_FACE ( 'NONE', ( #17066 ), #4491, .T. ) ;
#3213=AXIS2_PLACEMENT_3D ( 'NONE', #15612, #6977, #14222 ) ;
#3215=AXIS2_PLACEMENT_3D ( 'NONE', #7307, #5749, #181 ) ;
#3216=AXIS2_PLACEMENT_3D ( 'NONE', #10862, #13548, #6512 ) ;
#3221=FACE_OUTER_BOUND ( 'NONE', #16383, .T. ) ;
#3223=ORIENTED_EDGE ( 'NONE', *, *, #4672, .T. ) ;
#3226=ORIENTED_EDGE ( 'NONE', *, *, #12932, .T. ) ;
#3227=CIRCLE ( 'NONE', #1748, 8.000000000000003553 ) ;
#3231=DIRECTION ( 'NONE',  ( 0.000000000000000000, 0.000000000000000000, 1.000000000000000000 ) ) ;
#3238=DIRECTION ( 'NONE',  ( 1.000000000000000000, 0.000000000000000000, -4.336808689942021680E-16 ) ) ;
#3242=LINE ( 'NONE', #3516, #4220 ) ;
#3251=DIRECTION ( 'NONE',  ( -3.373073425510457965E-16, 0.000000000000000000, -1.000000000000000000 ) ) ;
#3258=DIRECTION ( 'NONE',  ( 0.000000000000000000, 0.000000000000000000, 1.000000000000000000 ) ) ;
#3263=DIRECTION ( 'NONE',  ( -4.915049848600951133E-16, 0.000000000000000000, -1.000000000000000000 ) ) ;
#3267=AXIS2_PLACEMENT_3D ( 'NONE', #4851, #7621, #6338 ) ;
#3272=AXIS2_PLACEMENT_3D ( 'NONE', #4866, #10516, #13759 ) ;
#3276=EDGE_CURVE ( 'NONE', #16215, #8582, #9234, .T. ) ;
#3291=CARTESIAN_POINT ( 'NONE',  ( 10.00000000000000000, 43.00000000000000000, -2.500000000000003109 ) ) ;
#3299=DIRECTION ( 'NONE',  ( 1.000000000000000000, 0.000000000000000000, 0.000000000000000000 ) ) ;
#3303=DIRECTION ( 'NONE',  ( 3.469446951953612217E-16, -0.000000000000000000, 1.000000000000000000 ) ) ;
#3313=EDGE_LOOP ( 'NONE', ( #5304, #9111, #889, #9369 ) ) ;
#3319=DIRECTION ( 'NONE',  ( 0.000000000000000000, 0.000000000000000000, -1.000000000000000000 ) ) ;
#3325=EDGE_CURVE ( 'NONE', #3191, #13521, #5103, .T. ) ;
#3330=AXIS2_PLACEMENT_3D ( 'NONE', #296, #5844, #2811 ) ;
#3331=CARTESIAN_POINT ( 'NONE',  ( 8.000000000000000000, 29.79999999999999716, -2.500000000000000888 ) ) ;
#3335=CARTESIAN_POINT ( 'NONE',  ( 10.00000000000000000, 29.79999999999999716, -2.500000000000003109 ) ) ;
#3343=EDGE_LOOP ( 'NONE', ( #4756, #16088, #10073, #5139 ) ) ;
#3345=DIRECTION ( 'NONE',  ( -3.373073425510457965E-16, 0.000000000000000000, -1.000000000000000000 ) ) ;
#3356=CIRCLE ( 'NONE', #13403, 0.9999999999999991118 ) ;
#3359=EDGE_LOOP ( 'NONE', ( #5671, #3956, #13155, #10290 ) ) ;
#3371=TOROIDAL_SURFACE ( 'NONE', #13719, 9.000000000000003553, 0.9999999999999991118 ) ;
#3372=FACE_OUTER_BOUND ( 'NONE', #11938, .T. ) ;
#3373=CARTESIAN_POINT ( 'NONE',  ( -9.000000000000001776, 34.19999999999999574, 2.499999999999998224 ) ) ;
#3388=DIRECTION ( 'NONE',  ( -0.000000000000000000, -1.000000000000000000, -0.000000000000000000 ) ) ;
#3389=DIRECTION ( 'NONE',  ( 0.000000000000000000, 0.000000000000000000, -1.000000000000000000 ) ) ;
#3395=CARTESIAN_POINT ( 'NONE',  ( 8.000000000000005329, 31.99999999999999289, 2.499999999999997780 ) ) ;
#3397=CARTESIAN_POINT ( 'NONE',  ( 0.000000000000000000, 20.99999999999999289, 2.500000000000000000 ) ) ;
#3400=EDGE_CURVE ( 'NONE', #3107, #13234, #13337, .T. ) ;
#3406=DIRECTION ( 'NONE',  ( -0.000000000000000000, -1.000000000000000000, -0.000000000000000000 ) ) ;
#3418=DIRECTION ( 'NONE',  ( 0.000000000000000000, 0.000000000000000000, -1.000000000000000000 ) ) ;
#3422=DIRECTION ( 'NONE',  ( -0.000000000000000000, -1.000000000000000000, -0.000000000000000000 ) ) ;
#3424=CARTESIAN_POINT ( 'NONE',  ( -1.734723475976807094E-15, 20.99999999999999289, -2.500000000000000000 ) ) ;
#3427=DIRECTION ( 'NONE',  ( 3.469446951953612217E-16, -0.000000000000000000, 1.000000000000000000 ) ) ;
#3432=ORIENTED_EDGE ( 'NONE', *, *, #2173, .F. ) ;
#3449=VERTEX_POINT ( 'NONE', #648 ) ;
#3464=ORIENTED_EDGE ( 'NONE', *, *, #16720, .T. ) ;
#3465=EDGE_LOOP ( 'NONE', ( #16428, #11013, #9702, #13555 ) ) ;
#3466=APPLICATION_CONTEXT ( 'automotive_design' ) ;
#3470=VERTEX_POINT ( 'NONE', #17638 ) ;
#3472=AXIS2_PLACEMENT_3D ( 'NONE', #4111, #5323, #18146 ) ;
#3475=CARTESIAN_POINT ( 'NONE',  ( 9.999999999999998224, 34.19999999999999574, -2.500000000000001776 ) ) ;
#3478=TOROIDAL_SURFACE ( 'NONE', #5832, 9.000000000000001776, 0.9999999999999991118 ) ;
#3491=CIRCLE ( 'NONE', #6735, 8.000000000000001776 ) ;
#3493=AXIS2_PLACEMENT_3D ( 'NONE', #9128, #14620, #14808 ) ;
#3495=ORIENTED_EDGE ( 'NONE', *, *, #8063, .T. ) ;
#3499=EDGE_LOOP ( 'NONE', ( #10498, #8414, #3226, #10524 ) ) ;
#3500=EDGE_CURVE ( 'NONE', #10466, #15990, #15193, .T. ) ;
#3501=CARTESIAN_POINT ( 'NONE',  ( 8.000000000000005329, 20.99999999999999289, 2.499999999999997780 ) ) ;
#3505=CARTESIAN_POINT ( 'NONE',  ( 9.999999999999998224, 20.99999999999999289, -2.500000000000001776 ) ) ;
#3506=ADVANCED_FACE ( 'NONE', ( #17722 ), #17580, .T. ) ;
#3507=TOROIDAL_SURFACE ( 'NONE', #16559, 9.000000000000001776, 0.9999999999999991118 ) ;
#3513=EDGE_LOOP ( 'NONE', ( #4686, #17563, #7440, #5711 ) ) ;
#3514=EDGE_LOOP ( 'NONE', ( #12299, #6468, #2485, #7809 ) ) ;
#3516=CARTESIAN_POINT ( 'NONE',  ( 8.000000000000001776, 29.79999999999999716, -2.500000000000002220 ) ) ;
#3520=ORIENTED_EDGE ( 'NONE', *, *, #2483, .T. ) ;
#3523=TOROIDAL_SURFACE ( 'NONE', #13576, 9.000000000000001776, 0.9999999999999991118 ) ;
#3535=AXIS2_PLACEMENT_3D ( 'NONE', #6208, #14946, #4627 ) ;
#3543=CARTESIAN_POINT ( 'NONE',  ( -9.000000000000001776, 38.59999999999999432, 2.499999999999998224 ) ) ;
#3553=DIRECTION ( 'NONE',  ( -0.000000000000000000, -1.000000000000000000, -0.000000000000000000 ) ) ;
#3554=CIRCLE ( 'NONE', #6511, 8.000000000000001776 ) ;
#3555=DIRECTION ( 'NONE',  ( 0.000000000000000000, 0.000000000000000000, -1.000000000000000000 ) ) ;
#3563=TOROIDAL_SURFACE ( 'NONE', #11843, 9.000000000000001776, 0.9999999999999991118 ) ;
#3568=CARTESIAN_POINT ( 'NONE',  ( -9.000000000000001776, 43.00000000000000000, 2.499999999999998224 ) ) ;
#3570=TOROIDAL_SURFACE ( 'NONE', #13641, 9.000000000000001776, 0.9999999999999991118 ) ;
#3572=DIRECTION ( 'NONE',  ( 0.000000000000000000, 0.000000000000000000, 1.000000000000000000 ) ) ;
#3588=DIRECTION ( 'NONE',  ( -0.000000000000000000, -1.000000000000000000, -0.000000000000000000 ) ) ;
#3589=DIRECTION ( 'NONE',  ( 0.000000000000000000, 0.000000000000000000, -1.000000000000000000 ) ) ;
#3595=ORIENTED_EDGE ( 'NONE', *, *, #17528, .T. ) ;
#3599=ORIENTED_EDGE ( 'NONE', *, *, #13575, .F. ) ;
#3600=DIRECTION ( 'NONE',  ( 0.000000000000000000, 0.000000000000000000, -1.000000000000000000 ) ) ;
#3603=CIRCLE ( 'NONE', #13068, 0.9999999999999991118 ) ;
#3605=EDGE_CURVE ( 'NONE', #1028, #10466, #8630, .T. ) ;
#3607=ORIENTED_EDGE ( 'NONE', *, *, #6701, .T. ) ;
#3611=ORIENTED_EDGE ( 'NONE', *, *, #13294, .F. ) ;
#3615=AXIS2_PLACEMENT_3D ( 'NONE', #16001, #8933, #13198 ) ;
#3617=( GEOMETRIC_REPRESENTATION_CONTEXT ( 3 ) GLOBAL_UNCERTAINTY_ASSIGNED_CONTEXT ( ( #16777 ) ) GLOBAL_UNIT_ASSIGNED_CONTEXT ( ( #5096, #13720, #1031 ) ) REPRESENTATION_CONTEXT ( 'NONE', 'WORKASPACE' ) );
#3622=ADVANCED_FACE ( 'NONE', ( #6739 ), #2751, .T. ) ;
#3638=ORIENTED_EDGE ( 'NONE', *, *, #16368, .F. ) ;
#3644=AXIS2_PLACEMENT_3D ( 'NONE', #12887, #14108, #193 ) ;
#3646=ORIENTED_EDGE ( 'NONE', *, *, #18354, .F. ) ;
#3647=CYLINDRICAL_SURFACE ( 'NONE', #608, 0.9999999999999991118 ) ;
#3649=VERTEX_POINT ( 'NONE', #5354 ) ;
#3655=CIRCLE ( 'NONE', #9860, 0.9999999999999991118 ) ;
#3667=VERTEX_POINT ( 'NONE', #16775 ) ;
#3669=AXIS2_PLACEMENT_3D ( 'NONE', #3568, #10221, #4576 ) ;
#3670=ADVANCED_FACE ( 'NONE', ( #4044 ), #3928, .T. ) ;
#3672=ORIENTED_EDGE ( 'NONE', *, *, #7203, .T. ) ;
#3677=ORIENTED_EDGE ( 'NONE', *, *, #13039, .F. ) ;
#3691=ORIENTED_EDGE ( 'NONE', *, *, #10633, .F. ) ;
#3697=ORIENTED_EDGE ( 'NONE', *, *, #1178, .T. ) ;
#3701=CARTESIAN_POINT ( 'NONE',  ( 9.000000000000005329, 40.79999999999999716, 2.499999999999997335 ) ) ;
#3703=CARTESIAN_POINT ( 'NONE',  ( -1.734723475976807094E-15, 34.19999999999999574, -12.50000000000000000 ) ) ;
#3706=DIRECTION ( 'NONE',  ( 0.000000000000000000, 0.000000000000000000, -1.000000000000000000 ) ) ;
#3719=VERTEX_POINT ( 'NONE', #16867 ) ;
#3723=EDGE_CURVE ( 'NONE', #11211, #5374, #5399, .T. ) ;
#3724=TOROIDAL_SURFACE ( 'NONE', #2842, 9.000000000000001776, 0.9999999999999991118 ) ;
#3733=ORIENTED_EDGE ( 'NONE', *, *, #10684, .F. ) ;
#3738=AXIS2_PLACEMENT_3D ( 'NONE', #1055, #2452, #16546 ) ;
#3745=CARTESIAN_POINT ( 'NONE',  ( 9.000000000000001776, 34.19999999999999574, -2.500000000000002665 ) ) ;
#3746=CIRCLE ( 'NONE', #11719, 0.9999999999999991118 ) ;
#3753=CARTESIAN_POINT ( 'NONE',  ( 9.000000000000000000, 40.79999999999999716, -2.500000000000001332 ) ) ;
#3755=CARTESIAN_POINT ( 'NONE',  ( 0.000000000000000000, 25.39999999999999503, 2.500000000000000000 ) ) ;
#3758=FACE_OUTER_BOUND ( 'NONE', #268, .T. ) ;
#3759=ADVANCED_FACE ( 'NONE', ( #2939 ), #5626, .T. ) ;
#3776=ORIENTED_EDGE ( 'NONE', *, *, #17630, .F. ) ;
#3783=VERTEX_POINT ( 'NONE', #12664 ) ;
#3788=AXIS2_PLACEMENT_3D ( 'NONE', #6165, #4773, #17224 ) ;
#3789=DIRECTION ( 'NONE',  ( 1.000000000000000000, 0.000000000000000000, 0.000000000000000000 ) ) ;
#3794=ORIENTED_EDGE ( 'NONE', *, *, #16427, .F. ) ;
#3809=CARTESIAN_POINT ( 'NONE',  ( -9.000000000000003553, 25.39999999999999503, -2.500000000000001776 ) ) ;
#3811=FACE_OUTER_BOUND ( 'NONE', #3853, .T. ) ;
#3817=CYLINDRICAL_SURFACE ( 'NONE', #18336, 0.9999999999999991118 ) ;
#3822=EDGE_CURVE ( 'NONE', #5909, #6012, #6302, .T. ) ;
#3825=EDGE_LOOP ( 'NONE', ( #4853, #15736, #14077, #7623 ) ) ;
#3829=EDGE_CURVE ( 'NONE', #17541, #1681, #6285, .T. ) ;
#3830=AXIS2_PLACEMENT_3D ( 'NONE', #13961, #15187, #1274 ) ;
#3833=TOROIDAL_SURFACE ( 'NONE', #18362, 9.000000000000001776, 0.9999999999999991118 ) ;
#3834=ADVANCED_FACE ( 'NONE', ( #14058 ), #16372, .T. ) ;
#3835=CARTESIAN_POINT ( 'NONE',  ( -9.000000000000003553, 20.99999999999999289, -2.500000000000001776 ) ) ;
#3840=AXIS2_PLACEMENT_3D ( 'NONE', #4204, #14033, #15527 ) ;
#3842=DIRECTION ( 'NONE',  ( -1.000000000000000000, 0.000000000000000000, 0.000000000000000000 ) ) ;
#3849=DIRECTION ( 'NONE',  ( 1.000000000000000000, 0.000000000000000000, 0.000000000000000000 ) ) ;
#3853=EDGE_LOOP ( 'NONE', ( #17157, #18021, #8464, #5830 ) ) ;
#3855=AXIS2_PLACEMENT_3D ( 'NONE', #1522, #1610, #4379 ) ;
#3861=DIRECTION ( 'NONE',  ( -3.373073425510457965E-16, 0.000000000000000000, -1.000000000000000000 ) ) ;
#3862=DIRECTION ( 'NONE',  ( 0.000000000000000000, 0.000000000000000000, -1.000000000000000000 ) ) ;
#3871=EDGE_LOOP ( 'NONE', ( #9992, #15272, #1948, #15222 ) ) ;
#3872=DIRECTION ( 'NONE',  ( -0.000000000000000000, -1.000000000000000000, -0.000000000000000000 ) ) ;
#3873=( LENGTH_UNIT ( ) NAMED_UNIT ( * ) SI_UNIT ( .MILLI., .METRE. ) );
#3875=CARTESIAN_POINT ( 'NONE',  ( 8.000000000000005329, 27.59999999999999432, 2.499999999999997780 ) ) ;
#3890=DIRECTION ( 'NONE',  ( 1.000000000000000000, 0.000000000000000000, 0.000000000000000000 ) ) ;
#3897=CIRCLE ( 'NONE', #654, 10.00000000000000178 ) ;
#3910=DIRECTION ( 'NONE',  ( 0.000000000000000000, 0.000000000000000000, 1.000000000000000000 ) ) ;
#3913=ORIENTED_EDGE ( 'NONE', *, *, #4609, .F. ) ;
#3919=VERTEX_POINT ( 'NONE', #14912 ) ;
#3928=TOROIDAL_SURFACE ( 'NONE', #14594, 9.000000000000003553, 0.9999999999999991118 ) ;
#3937=FACE_OUTER_BOUND ( 'NONE', #2867, .T. ) ;
#3939=CARTESIAN_POINT ( 'NONE',  ( -1.734723475976807094E-15, 23.19999999999999574, -11.50000000000000178 ) ) ;
#3949=DIRECTION ( 'NONE',  ( 0.000000000000000000, 0.000000000000000000, 1.000000000000000000 ) ) ;
#3951=CIRCLE ( 'NONE', #709, 10.00000000000000000 ) ;
#3956=ORIENTED_EDGE ( 'NONE', *, *, #15559, .T. ) ;
#3957=CARTESIAN_POINT ( 'NONE',  ( 8.000000000000005329, 29.79999999999999716, 2.499999999999997780 ) ) ;
#3960=ORIENTED_EDGE ( 'NONE', *, *, #9531, .T. ) ;
#3966=AXIS2_PLACEMENT_3D ( 'NONE', #10127, #8735, #606 ) ;
#3972=FACE_OUTER_BOUND ( 'NONE', #11222, .T. ) ;
#3974=DIRECTION ( 'NONE',  ( -1.000000000000000000, 0.000000000000000000, 4.336808689942021680E-16 ) ) ;
#3978=DIRECTION ( 'NONE',  ( 1.000000000000000000, 0.000000000000000000, 0.000000000000000000 ) ) ;
#3984=ORIENTED_EDGE ( 'NONE', *, *, #16350, .F. ) ;
#3989=EDGE_CURVE ( 'NONE', #4032, #3136, #1932, .T. ) ;
#3992=ADVANCED_FACE ( 'NONE', ( #10241 ), #16112, .T. ) ;
#4002=CARTESIAN_POINT ( 'NONE',  ( 9.000000000000005329, 20.99999999999999289, 2.499999999999997335 ) ) ;
#4003=DIRECTION ( 'NONE',  ( -1.000000000000000000, 0.000000000000000000, 4.336808689942021680E-16 ) ) ;
#4004=ORIENTED_EDGE ( 'NONE', *, *, #15347, .F. ) ;
#4005=ORIENTED_EDGE ( 'NONE', *, *, #7028, .T. ) ;
#4021=DIRECTION ( 'NONE',  ( 1.000000000000000000, 0.000000000000000000, 0.000000000000000000 ) ) ;
#4026=( NAMED_UNIT ( * ) PLANE_ANGLE_UNIT ( ) SI_UNIT ( $, .RADIAN. ) );
#4031=CARTESIAN_POINT ( 'NONE',  ( 0.000000000000000000, 40.79999999999999716, 2.500000000000000000 ) ) ;
#4032=VERTEX_POINT ( 'NONE', #14533 ) ;
#4037=CYLINDRICAL_SURFACE ( 'NONE', #15400, 0.9999999999999991118 ) ;
#4040=ORIENTED_EDGE ( 'NONE', *, *, #1119, .T. ) ;
#4044=FACE_OUTER_BOUND ( 'NONE', #4802, .T. ) ;
#4048=AXIS2_PLACEMENT_3D ( 'NONE', #13090, #406, #4652 ) ;
#4058=( NAMED_UNIT ( * ) PLANE_ANGLE_UNIT ( ) SI_UNIT ( $, .RADIAN. ) );
#4059=CARTESIAN_POINT ( 'NONE',  ( 8.000000000000005329, 18.79999999999999361, 2.499999999999997780 ) ) ;
#4061=DIRECTION ( 'NONE',  ( 0.000000000000000000, 0.000000000000000000, 1.000000000000000000 ) ) ;
#4064=EDGE_LOOP ( 'NONE', ( #3599, #15378, #2449, #12860 ) ) ;
#4087=AXIS2_PLACEMENT_3D ( 'NONE', #5491, #11314, #13932 ) ;
#4090=CIRCLE ( 'NONE', #3215, 0.9999999999999991118 ) ;
#4091=ORIENTED_EDGE ( 'NONE', *, *, #11924, .F. ) ;
#4097=CARTESIAN_POINT ( 'NONE',  ( -9.000000000000001776, 25.39999999999999503, 2.499999999999995559 ) ) ;
#4099=ORIENTED_EDGE ( 'NONE', *, *, #15232, .F. ) ;
#4106=MECHANICAL_DESIGN_GEOMETRIC_PRESENTATION_REPRESENTATION('',(#5592),#4682);
#4111=CARTESIAN_POINT ( 'NONE',  ( 9.000000000000000000, 18.79999999999999361, -2.500000000000001332 ) ) ;
#4112=ADVANCED_FACE ( 'NONE', ( #16756 ), #12190, .T. ) ;
#4115=ADVANCED_FACE ( 'NONE', ( #2386 ), #990, .T. ) ;
#4126=DIRECTION ( 'NONE',  ( 0.000000000000000000, 0.000000000000000000, 1.000000000000000000 ) ) ;
#4128=CIRCLE ( 'NONE', #16880, 0.9999999999999991118 ) ;
#4132=AXIS2_PLACEMENT_3D ( 'NONE', #18368, #4249, #18101 ) ;
#4133=DIRECTION ( 'NONE',  ( -0.000000000000000000, -1.000000000000000000, -0.000000000000000000 ) ) ;
#4134=DIRECTION ( 'NONE',  ( -0.000000000000000000, -1.000000000000000000, -0.000000000000000000 ) ) ;
#4142=EDGE_LOOP ( 'NONE', ( #14105, #3638, #12025, #940 ) ) ;
#4150=EDGE_LOOP ( 'NONE', ( #13636, #4005, #4634, #13466 ) ) ;
#4153=ORIENTED_EDGE ( 'NONE', *, *, #10556, .F. ) ;
#4155=CARTESIAN_POINT ( 'NONE',  ( -8.000000000000001776, 20.99999999999999289, 2.499999999999998224 ) ) ;
#4161=VERTEX_POINT ( 'NONE', #9319 ) ;
#4163=LINE ( 'NONE', #12318, #2355 ) ;
#4164=ADVANCED_FACE ( 'NONE', ( #10892 ), #14612, .T. ) ;
#4165=VERTEX_POINT ( 'NONE', #2478 ) ;
#4168=EDGE_CURVE ( 'NONE', #16215, #3649, #17597, .T. ) ;
#4169=CARTESIAN_POINT ( 'NONE',  ( -10.00000000000000178, 34.19999999999999574, -2.500000000000001776 ) ) ;
#4174=AXIS2_PLACEMENT_3D ( 'NONE', #13691, #5620, #9786 ) ;
#4177=EDGE_LOOP ( 'NONE', ( #11943, #1017, #253, #9566 ) ) ;
#4186=ORIENTED_EDGE ( 'NONE', *, *, #7385, .T. ) ;
#4199=LINE ( 'NONE', #17100, #2276 ) ;
#4204=CARTESIAN_POINT ( 'NONE',  ( -9.000000000000001776, 43.00000000000000000, 2.499999999999995559 ) ) ;
#4217=AXIS2_PLACEMENT_3D ( 'NONE', #16498, #3872, #2316 ) ;
#4220=VECTOR ( 'NONE', #4530, 1000.000000000000000 ) ;
#4221=EDGE_CURVE ( 'NONE', #17692, #5913, #3356, .T. ) ;
#4226=EDGE_CURVE ( 'NONE', #8512, #5725, #7478, .T. ) ;
#4228=FACE_OUTER_BOUND ( 'NONE', #7273, .T. ) ;
#4232=AXIS2_PLACEMENT_3D ( 'NONE', #5196, #9187, #14773 ) ;
#4238=CARTESIAN_POINT ( 'NONE',  ( -1.734723475976807094E-15, 23.19999999999999574, -2.500000000000000000 ) ) ;
#4245=EDGE_LOOP ( 'NONE', ( #5453, #9525, #15281, #3672 ) ) ;
#4249=DIRECTION ( 'NONE',  ( 0.000000000000000000, 0.000000000000000000, 1.000000000000000000 ) ) ;
#4251=ORIENTED_EDGE ( 'NONE', *, *, #5422, .F. ) ;
#4252=CARTESIAN_POINT ( 'NONE',  ( -9.000000000000001776, 40.79999999999999716, 2.499999999999998224 ) ) ;
#4256=TOROIDAL_SURFACE ( 'NONE', #14941, 9.000000000000003553, 0.9999999999999991118 ) ;
#4264=TOROIDAL_SURFACE ( 'NONE', #16745, 9.000000000000001776, 0.9999999999999991118 ) ;
#4277=DIRECTION ( 'NONE',  ( -0.000000000000000000, -1.000000000000000000, -0.000000000000000000 ) ) ;
#4296=ORIENTED_EDGE ( 'NONE', *, *, #15457, .F. ) ;
#4307=CARTESIAN_POINT ( 'NONE',  ( -8.000000000000001776, 40.79999999999999716, 2.499999999999998224 ) ) ;
#4310=CIRCLE ( 'NONE', #14706, 0.9999999999999991118 ) ;
#4316=EDGE_CURVE ( 'NONE', #12374, #5212, #13708, .T. ) ;
#4317=ORIENTED_EDGE ( 'NONE', *, *, #8030, .F. ) ;
#4318=CARTESIAN_POINT ( 'NONE',  ( 9.000000000000000000, 43.00000000000000000, -2.500000000000001332 ) ) ;
#4326=AXIS2_PLACEMENT_3D ( 'NONE', #14237, #8209, #9605 ) ;
#4328=DIRECTION ( 'NONE',  ( 0.000000000000000000, 0.000000000000000000, 1.000000000000000000 ) ) ;
#4331=CARTESIAN_POINT ( 'NONE',  ( -1.734723475976807094E-15, 40.79999999999999716, -2.500000000000000000 ) ) ;
#4338=CIRCLE ( 'NONE', #14117, 0.9999999999999991118 ) ;
#4356=CARTESIAN_POINT ( 'NONE',  ( -1.734723475976807094E-15, 36.39999999999999147, -2.500000000000000000 ) ) ;
#4362=ORIENTED_EDGE ( 'NONE', *, *, #18253, .T. ) ;
#4363=( GEOMETRIC_REPRESENTATION_CONTEXT ( 3 ) GLOBAL_UNCERTAINTY_ASSIGNED_CONTEXT ( ( #2502 ) ) GLOBAL_UNIT_ASSIGNED_CONTEXT ( ( #4384, #2914, #124 ) ) REPRESENTATION_CONTEXT ( 'NONE', 'WORKASPACE' ) );
#4369=CARTESIAN_POINT ( 'NONE',  ( 0.000000000000000000, 23.19999999999999574, 2.500000000000000000 ) ) ;
#4373=CIRCLE ( 'NONE', #18342, 0.9999999999999991118 ) ;
#4376=AXIS2_PLACEMENT_3D ( 'NONE', #11978, #10496, #3555 ) ;
#4379=DIRECTION ( 'NONE',  ( 0.000000000000000000, 0.000000000000000000, 1.000000000000000000 ) ) ;
#4384=( LENGTH_UNIT ( ) NAMED_UNIT ( * ) SI_UNIT ( .MILLI., .METRE. ) );
#4387=EDGE_CURVE ( 'NONE', #12622, #11211, #16679, .T. ) ;
#4388=DIRECTION ( 'NONE',  ( 0.000000000000000000, 0.000000000000000000, 1.000000000000000000 ) ) ;
#4390=ADVANCED_FACE ( 'NONE', ( #17750 ), #12221, .T. ) ;
#4394=CIRCLE ( 'NONE', #13875, 0.9999999999999991118 ) ;
#4395=CARTESIAN_POINT ( 'NONE',  ( 8.000000000000000000, 16.59999999999999787, -2.500000000000000888 ) ) ;
#4400=DIRECTION ( 'NONE',  ( 3.469446951953612217E-16, -0.000000000000000000, 1.000000000000000000 ) ) ;
#4403=AXIS2_PLACEMENT_3D ( 'NONE', #2860, #5729, #3974 ) ;
#4412=CARTESIAN_POINT ( 'NONE',  ( -9.000000000000001776, 38.59999999999999432, 2.499999999999995559 ) ) ;
#4414=CARTESIAN_POINT ( 'NONE',  ( -10.00000000000000000, 43.00000000000000000, 2.499999999999996003 ) ) ;
#4423=EDGE_CURVE ( 'NONE', #13234, #17672, #12513, .T. ) ;
#4426=CARTESIAN_POINT ( 'NONE',  ( 10.00000000000000000, 23.19999999999999574, -2.500000000000003109 ) ) ;
#4432=ORIENTED_EDGE ( 'NONE', *, *, #10855, .F. ) ;
#4440=ORIENTED_EDGE ( 'NONE', *, *, #14899, .T. ) ;
#4446=DIRECTION ( 'NONE',  ( 0.000000000000000000, 0.000000000000000000, 1.000000000000000000 ) ) ;
#4447=EDGE_CURVE ( 'NONE', #12413, #3919, #6601, .T. ) ;
#4453=EDGE_CURVE ( 'NONE', #3783, #634, #15210, .T. ) ;
#4455=ORIENTED_EDGE ( 'NONE', *, *, #12935, .T. ) ;
#4456=EDGE_LOOP ( 'NONE', ( #10504, #7192, #11581, #5924 ) ) ;
#4461=ORIENTED_EDGE ( 'NONE', *, *, #1895, .T. ) ;
#4470=DIRECTION ( 'NONE',  ( 3.469446951953612217E-16, -0.000000000000000000, 1.000000000000000000 ) ) ;
#4471=CIRCLE ( 'NONE', #1531, 0.9999999999999991118 ) ;
#4481=DIRECTION ( 'NONE',  ( -0.000000000000000000, -1.000000000000000000, -0.000000000000000000 ) ) ;
#4485=AXIS2_PLACEMENT_3D ( 'NONE', #14640, #3588, #11928 ) ;
#4486=DIRECTION ( 'NONE',  ( 0.000000000000000000, 0.000000000000000000, 1.000000000000000000 ) ) ;
#4491=TOROIDAL_SURFACE ( 'NONE', #6862, 9.000000000000001776, 0.9999999999999991118 ) ;
#4495=EDGE_CURVE ( 'NONE', #12374, #11611, #583, .T. ) ;
#4498=DIRECTION ( 'NONE',  ( 1.000000000000000000, 0.000000000000000000, 0.000000000000000000 ) ) ;
#4508=CARTESIAN_POINT ( 'NONE',  ( -9.000000000000003553, 31.99999999999999289, -2.500000000000001776 ) ) ;
#4510=ORIENTED_EDGE ( 'NONE', *, *, #13407, .T. ) ;
#4516=DIRECTION ( 'NONE',  ( 1.000000000000000000, 0.000000000000000000, 0.000000000000000000 ) ) ;
#4519=AXIS2_PLACEMENT_3D ( 'NONE', #12054, #10760, #2163 ) ;
#4521=AXIS2_PLACEMENT_3D ( 'NONE', #7021, #6939, #11202 ) ;
#4522=FACE_OUTER_BOUND ( 'NONE', #12486, .T. ) ;
#4526=CYLINDRICAL_SURFACE ( 'NONE', #8493, 0.9999999999999991118 ) ;
#4527=ORIENTED_EDGE ( 'NONE', *, *, #16722, .F. ) ;
#4530=DIRECTION ( 'NONE',  ( 3.469446951953612217E-16, -0.000000000000000000, 1.000000000000000000 ) ) ;
#4534=AXIS2_PLACEMENT_3D ( 'NONE', #4508, #5985, #3034 ) ;
#4540=CARTESIAN_POINT ( 'NONE',  ( 0.000000000000000000, 36.39999999999999147, 2.500000000000000000 ) ) ;
#4545=VECTOR ( 'NONE', #10316, 1000.000000000000000 ) ;
#4547=VERTEX_POINT ( 'NONE', #7977 ) ;
#4551=EDGE_CURVE ( 'NONE', #11211, #16215, #4923, .T. ) ;
#4555=EDGE_CURVE ( 'NONE', #4719, #9180, #7182, .T. ) ;
#4567=ORIENTED_EDGE ( 'NONE', *, *, #16232, .T. ) ;
#4574=CARTESIAN_POINT ( 'NONE',  ( -9.000000000000003553, 16.59999999999999787, -2.500000000000001776 ) ) ;
#4575=CARTESIAN_POINT ( 'NONE',  ( -9.000000000000001776, 27.59999999999999432, 2.499999999999998224 ) ) ;
#4576=DIRECTION ( 'NONE',  ( 1.000000000000000000, 0.000000000000000000, 0.000000000000000000 ) ) ;
#4596=ORIENTED_EDGE ( 'NONE', *, *, #7843, .T. ) ;
#4599=ORIENTED_EDGE ( 'NONE', *, *, #12932, .F. ) ;
#4601=DIRECTION ( 'NONE',  ( -0.000000000000000000, -1.000000000000000000, -0.000000000000000000 ) ) ;
#4609=EDGE_CURVE ( 'NONE', #5374, #8582, #4899, .T. ) ;
#4611=DIRECTION ( 'NONE',  ( -3.469446951953613696E-16, -0.000000000000000000, -1.000000000000000000 ) ) ;
#4613=ORIENTED_EDGE ( 'NONE', *, *, #10319, .F. ) ;
#4627=DIRECTION ( 'NONE',  ( 0.000000000000000000, 0.000000000000000000, -1.000000000000000000 ) ) ;
#4631=AXIS2_PLACEMENT_3D ( 'NONE', #16370, #9150, #729 ) ;
#4634=ORIENTED_EDGE ( 'NONE', *, *, #12813, .T. ) ;
#4646=CIRCLE ( 'NONE', #11431, 0.9999999999999991118 ) ;
#4650=EDGE_CURVE ( 'NONE', #456, #2806, #6885, .T. ) ;
#4652=DIRECTION ( 'NONE',  ( 0.000000000000000000, 0.000000000000000000, -1.000000000000000000 ) ) ;
#4653=CARTESIAN_POINT ( 'NONE',  ( -10.00000000000000000, 16.59999999999999787, 2.499999999999996003 ) ) ;
#4654=VECTOR ( 'NONE', #10888, 1000.000000000000000 ) ;
#4655=FACE_OUTER_BOUND ( 'NONE', #15197, .T. ) ;
#4657=ORIENTED_EDGE ( 'NONE', *, *, #9303, .F. ) ;
#4672=EDGE_CURVE ( 'NONE', #9679, #6366, #6314, .T. ) ;
#4676=DIRECTION ( 'NONE',  ( 0.000000000000000000, 0.000000000000000000, 1.000000000000000000 ) ) ;
#4681=FACE_OUTER_BOUND ( 'NONE', #17306, .T. ) ;
#4682=( GEOMETRIC_REPRESENTATION_CONTEXT ( 3 ) GLOBAL_UNCERTAINTY_ASSIGNED_CONTEXT ( ( #1038 ) ) GLOBAL_UNIT_ASSIGNED_CONTEXT ( ( #1383, #4058, #12678 ) ) REPRESENTATION_CONTEXT ( 'NONE', 'WORKASPACE' ) );
#4685=AXIS2_PLACEMENT_3D ( 'NONE', #4934, #2178, #12340 ) ;
#4686=ORIENTED_EDGE ( 'NONE', *, *, #1178, .F. ) ;
#4696=( NAMED_UNIT ( * ) SI_UNIT ( $, .STERADIAN. ) SOLID_ANGLE_UNIT ( ) );
#4698=FACE_OUTER_BOUND ( 'NONE', #1877, .T. ) ;
#4705=ORIENTED_EDGE ( 'NONE', *, *, #10684, .T. ) ;
#4711=ORIENTED_EDGE ( 'NONE', *, *, #7028, .F. ) ;
#4719=VERTEX_POINT ( 'NONE', #3875 ) ;
#4723=CARTESIAN_POINT ( 'NONE',  ( 0.000000000000000000, 31.99999999999999289, 2.500000000000000000 ) ) ;
#4733=ORIENTED_EDGE ( 'NONE', *, *, #14526, .T. ) ;
#4746=DIRECTION ( 'NONE',  ( 3.469446951953612217E-16, -0.000000000000000000, 1.000000000000000000 ) ) ;
#4749=CARTESIAN_POINT ( 'NONE',  ( -1.734723475976807094E-15, 18.79999999999999361, -11.50000000000000178 ) ) ;
#4753=DIRECTION ( 'NONE',  ( 0.000000000000000000, 0.000000000000000000, -1.000000000000000000 ) ) ;
#4756=ORIENTED_EDGE ( 'NONE', *, *, #12726, .F. ) ;
#4765=CIRCLE ( 'NONE', #11266, 0.9999999999999991118 ) ;
#4773=DIRECTION ( 'NONE',  ( -0.000000000000000000, -1.000000000000000000, -0.000000000000000000 ) ) ;
#4775=CARTESIAN_POINT ( 'NONE',  ( -8.000000000000001776, 34.19999999999999574, 2.499999999999998224 ) ) ;
#4780=CARTESIAN_POINT ( 'NONE',  ( -10.00000000000000000, 27.59999999999999432, 2.499999999999996003 ) ) ;
#4781=EDGE_CURVE ( 'NONE', #1579, #1028, #3655, .T. ) ;
#4802=EDGE_LOOP ( 'NONE', ( #11395, #4440, #5564, #15802 ) ) ;
#4804=AXIS2_PLACEMENT_3D ( 'NONE', #18011, #6670, #9811 ) ;
#4806=AXIS2_PLACEMENT_3D ( 'NONE', #4097, #15514, #2726 ) ;
#4821=AXIS2_PLACEMENT_3D ( 'NONE', #827, #10733, #7767 ) ;
#4822=CARTESIAN_POINT ( 'NONE',  ( 10.00000000000000000, 40.79999999999999716, -2.500000000000003109 ) ) ;
#4827=MECHANICAL_DESIGN_GEOMETRIC_PRESENTATION_REPRESENTATION('',(#8072),#16407);
#4829=ORIENTED_EDGE ( 'NONE', *, *, #10457, .T. ) ;
#4835=AXIS2_PLACEMENT_3D ( 'NONE', #7415, #9087, #14767 ) ;
#4844=CARTESIAN_POINT ( 'NONE',  ( 0.000000000000000000, 29.79999999999999716, 2.500000000000000000 ) ) ;
#4848=DIRECTION ( 'NONE',  ( 0.000000000000000000, 0.000000000000000000, -1.000000000000000000 ) ) ;
#4851=CARTESIAN_POINT ( 'NONE',  ( -1.734723475976807094E-15, 25.39999999999999503, -11.50000000000000178 ) ) ;
#4853=ORIENTED_EDGE ( 'NONE', *, *, #11225, .F. ) ;
#4861=EDGE_CURVE ( 'NONE', #1681, #17541, #13416, .T. ) ;
#4866=CARTESIAN_POINT ( 'NONE',  ( -1.734723475976807094E-15, 25.39999999999999503, -2.500000000000000000 ) ) ;
#4871=DIRECTION ( 'NONE',  ( 3.469446951953612217E-16, -0.000000000000000000, 1.000000000000000000 ) ) ;
#4873=ORIENTED_EDGE ( 'NONE', *, *, #9442, .F. ) ;
#4878=EDGE_LOOP ( 'NONE', ( #12472, #9596, #7092, #1213 ) ) ;
#4886=FACE_OUTER_BOUND ( 'NONE', #18364, .T. ) ;
#4887=ADVANCED_FACE ( 'NONE', ( #3221 ), #15220, .T. ) ;
#4892=CARTESIAN_POINT ( 'NONE',  ( 8.000000000000005329, 38.59999999999999432, 2.499999999999997780 ) ) ;
#4899=LINE ( 'NONE', #15107, #14306 ) ;
#4901=TOROIDAL_SURFACE ( 'NONE', #15276, 9.000000000000003553, 0.9999999999999991118 ) ;
#4905=ORIENTED_EDGE ( 'NONE', *, *, #7189, .F. ) ;
#4911=EDGE_CURVE ( 'NONE', #11229, #6854, #17331, .T. ) ;
#4915=ORIENTED_EDGE ( 'NONE', *, *, #1923, .F. ) ;
#4921=VERTEX_POINT ( 'NONE', #15642 ) ;
#4923=LINE ( 'NONE', #9279, #10129 ) ;
#4932=CARTESIAN_POINT ( 'NONE',  ( 0.000000000000000000, 40.79999999999999716, 2.500000000000000000 ) ) ;
#4934=CARTESIAN_POINT ( 'NONE',  ( -9.000000000000003553, 29.79999999999999716, -2.500000000000001776 ) ) ;
#4935=ORIENTED_EDGE ( 'NONE', *, *, #1986, .F. ) ;
#4938=CARTESIAN_POINT ( 'NONE',  ( 9.000000000000001776, 29.79999999999999716, -2.500000000000002665 ) ) ;
#4940=ORIENTED_EDGE ( 'NONE', *, *, #14901, .T. ) ;
#4943=AXIS2_PLACEMENT_3D ( 'NONE', #2174, #10494, #16167 ) ;
#4949=EDGE_CURVE ( 'NONE', #1006, #13359, #15794, .T. ) ;
#4950=EDGE_CURVE ( 'NONE', #17672, #5212, #8671, .T. ) ;
#4955=EDGE_CURVE ( 'NONE', #2131, #12786, #8379, .T. ) ;
#4956=DIRECTION ( 'NONE',  ( 1.000000000000000000, 0.000000000000000000, -4.336808689942021680E-16 ) ) ;
#4958=DIRECTION ( 'NONE',  ( 0.000000000000000000, 0.000000000000000000, -1.000000000000000000 ) ) ;
#4978=EDGE_CURVE ( 'NONE', #11611, #1200, #3951, .T. ) ;
#4979=AXIS2_PLACEMENT_3D ( 'NONE', #6140, #15799, #311 ) ;
#4985=VERTEX_POINT ( 'NONE', #13314 ) ;
#4993=AXIS2_PLACEMENT_3D ( 'NONE', #11134, #10865, #11050 ) ;
#4995=CIRCLE ( 'NONE', #16826, 0.9999999999999991118 ) ;
#5004=TOROIDAL_SURFACE ( 'NONE', #16874, 9.000000000000001776, 0.9999999999999991118 ) ;
#5021=AXIS2_PLACEMENT_3D ( 'NONE', #13500, #14829, #17712 ) ;
#5026=FACE_OUTER_BOUND ( 'NONE', #8859, .T. ) ;
#5031=DIRECTION ( 'NONE',  ( -0.000000000000000000, -1.000000000000000000, -0.000000000000000000 ) ) ;
#5034=TOROIDAL_SURFACE ( 'NONE', #16003, 9.000000000000001776, 0.9999999999999991118 ) ;
#5039=FACE_OUTER_BOUND ( 'NONE', #6195, .T. ) ;
#5042=AXIS2_PLACEMENT_3D ( 'NONE', #8352, #16445, #16815 ) ;
#5045=CARTESIAN_POINT ( 'NONE',  ( -1.734723475976807094E-15, 43.00000000000000000, -11.50000000000000178 ) ) ;
#5062=EDGE_CURVE ( 'NONE', #5212, #13188, #628, .T. ) ;
#5066=AXIS2_PLACEMENT_3D ( 'NONE', #14716, #6259, #5140 ) ;
#5071=CARTESIAN_POINT ( 'NONE',  ( 9.000000000000005329, 38.59999999999999432, 2.499999999999997335 ) ) ;
#5084=ORIENTED_EDGE ( 'NONE', *, *, #12488, .F. ) ;
#5088=AXIS2_PLACEMENT_3D ( 'NONE', #6027, #7228, #7414 ) ;
#5090=AXIS2_PLACEMENT_3D ( 'NONE', #17657, #17373, #9183 ) ;
#5094=ORIENTED_EDGE ( 'NONE', *, *, #10488, .F. ) ;
#5096=( LENGTH_UNIT ( ) NAMED_UNIT ( * ) SI_UNIT ( .MILLI., .METRE. ) );
#5103=CIRCLE ( 'NONE', #2166, 0.9999999999999991118 ) ;
#5105=AXIS2_PLACEMENT_3D ( 'NONE', #7298, #10546, #8980 ) ;
#5112=ADVANCED_FACE ( 'NONE', ( #17522 ), #3371, .T. ) ;
#5117=EDGE_LOOP ( 'NONE', ( #6504, #7510, #6578, #4186 ) ) ;
#5126=EDGE_CURVE ( 'NONE', #2406, #6613, #16107, .T. ) ;
#5130=CIRCLE ( 'NONE', #7196, 8.000000000000001776 ) ;
#5139=ORIENTED_EDGE ( 'NONE', *, *, #141, .T. ) ;
#5140=DIRECTION ( 'NONE',  ( 0.000000000000000000, 0.000000000000000000, -1.000000000000000000 ) ) ;
#5142=CYLINDRICAL_SURFACE ( 'NONE', #7011, 0.9999999999999991118 ) ;
#5154=AXIS2_PLACEMENT_3D ( 'NONE', #3809, #8260, #9465 ) ;
#5156=CARTESIAN_POINT ( 'NONE',  ( -8.000000000000001776, 20.99999999999999289, 2.499999999999995115 ) ) ;
#5161=DIRECTION ( 'NONE',  ( -3.373073425510457965E-16, 0.000000000000000000, -1.000000000000000000 ) ) ;
#5164=CARTESIAN_POINT ( 'NONE',  ( 0.000000000000000000, 43.00000000000000000, 2.500000000000000000 ) ) ;
#5171=DIRECTION ( 'NONE',  ( -1.000000000000000000, 0.000000000000000000, 4.336808689942021680E-16 ) ) ;
#5189=FACE_OUTER_BOUND ( 'NONE', #13823, .T. ) ;
#5191=CARTESIAN_POINT ( 'NONE',  ( -1.734723475976807094E-15, 18.79999999999999361, -12.50000000000000000 ) ) ;
#5195=ADVANCED_FACE ( 'NONE', ( #3758 ), #8110, .T. ) ;
#5196=CARTESIAN_POINT ( 'NONE',  ( -1.734723475976807094E-15, 20.99999999999999289, -2.500000000000000000 ) ) ;
#5206=( NAMED_UNIT ( * ) PLANE_ANGLE_UNIT ( ) SI_UNIT ( $, .RADIAN. ) );
#5209=FACE_OUTER_BOUND ( 'NONE', #10320, .T. ) ;
#5212=VERTEX_POINT ( 'NONE', #9678 ) ;
#5222=AXIS2_PLACEMENT_3D ( 'NONE', #139, #9955, #12836 ) ;
#5225=ADVANCED_FACE ( 'NONE', ( #9320 ), #2491, .T. ) ;
#5237=DIRECTION ( 'NONE',  ( 3.469446951953612217E-16, -0.000000000000000000, 1.000000000000000000 ) ) ;
#5245=AXIS2_PLACEMENT_3D ( 'NONE', #5344, #5161, #6822 ) ;
#5255=DIRECTION ( 'NONE',  ( -1.000000000000000000, 0.000000000000000000, 4.336808689942021680E-16 ) ) ;
#5259=EDGE_LOOP ( 'NONE', ( #8572, #1053, #8322, #8785 ) ) ;
#5267=ORIENTED_EDGE ( 'NONE', *, *, #14835, .T. ) ;
#5274=DIRECTION ( 'NONE',  ( -3.373073425510457965E-16, 0.000000000000000000, -1.000000000000000000 ) ) ;
#5278=DIRECTION ( 'NONE',  ( 0.000000000000000000, 0.000000000000000000, 1.000000000000000000 ) ) ;
#5282=DIRECTION ( 'NONE',  ( -4.915049848600951133E-16, 0.000000000000000000, -1.000000000000000000 ) ) ;
#5284=MECHANICAL_DESIGN_GEOMETRIC_PRESENTATION_REPRESENTATION('',(#9417),#2050);
#5294=EDGE_CURVE ( 'NONE', #15972, #1567, #5130, .T. ) ;
#5299=AXIS2_PLACEMENT_3D ( 'NONE', #10252, #14641, #1560 ) ;
#5304=ORIENTED_EDGE ( 'NONE', *, *, #9531, .F. ) ;
#5316=AXIS2_PLACEMENT_3D ( 'NONE', #17534, #7479, #13227 ) ;
#5320=CARTESIAN_POINT ( 'NONE',  ( -9.000000000000001776, 40.79999999999999716, 2.499999999999995559 ) ) ;
#5323=DIRECTION ( 'NONE',  ( -3.373073425510457965E-16, 0.000000000000000000, -1.000000000000000000 ) ) ;
#5325=VECTOR ( 'NONE', #12269, 1000.000000000000000 ) ;
#5326=CARTESIAN_POINT ( 'NONE',  ( 9.000000000000005329, 16.59999999999999787, 2.499999999999997335 ) ) ;
#5328=FACE_OUTER_BOUND ( 'NONE', #14739, .T. ) ;
#5331=CARTESIAN_POINT ( 'NONE',  ( 0.000000000000000000, 43.00000000000000000, 2.500000000000000000 ) ) ;
#5342=DIRECTION ( 'NONE',  ( 1.000000000000000000, 0.000000000000000000, 0.000000000000000000 ) ) ;
#5343=CARTESIAN_POINT ( 'NONE',  ( -8.000000000000001776, 25.39999999999999503, 2.499999999999995115 ) ) ;
#5344=CARTESIAN_POINT ( 'NONE',  ( 9.000000000000000000, 27.59999999999999432, -2.500000000000001332 ) ) ;
#5347=EDGE_LOOP ( 'NONE', ( #2498, #14004, #148, #5582 ) ) ;
#5350=AXIS2_PLACEMENT_3D ( 'NONE', #13783, #11172, #18257 ) ;
#5352=EDGE_CURVE ( 'NONE', #11426, #4161, #1619, .T. ) ;
#5354=CARTESIAN_POINT ( 'NONE',  ( -8.000000000000001776, 25.39999999999999503, 2.499999999999998224 ) ) ;
#5357=EDGE_CURVE ( 'NONE', #15102, #5921, #13432, .T. ) ;
#5359=DIRECTION ( 'NONE',  ( -3.373073425510457965E-16, 0.000000000000000000, -1.000000000000000000 ) ) ;
#5367=VECTOR ( 'NONE', #12183, 1000.000000000000000 ) ;
#5370=DIRECTION ( 'NONE',  ( 0.000000000000000000, 0.000000000000000000, -1.000000000000000000 ) ) ;
#5374=VERTEX_POINT ( 'NONE', #8553 ) ;
#5379=( GEOMETRIC_REPRESENTATION_CONTEXT ( 3 ) GLOBAL_UNCERTAINTY_ASSIGNED_CONTEXT ( ( #8113 ) ) GLOBAL_UNIT_ASSIGNED_CONTEXT ( ( #13700, #742, #6385 ) ) REPRESENTATION_CONTEXT ( 'NONE', 'WORKASPACE' ) );
#5399=CIRCLE ( 'NONE', #676, 0.9999999999999991118 ) ;
#5402=ORIENTED_EDGE ( 'NONE', *, *, #1921, .T. ) ;
#5410=CARTESIAN_POINT ( 'NONE',  ( -1.734723475976807094E-15, 34.19999999999999574, -2.500000000000000000 ) ) ;
#5411=STYLED_ITEM('',(#18396),#8199);
#5420=( LENGTH_UNIT ( ) NAMED_UNIT ( * ) SI_UNIT ( .MILLI., .METRE. ) );
#5422=EDGE_CURVE ( 'NONE', #2131, #9627, #5434, .T. ) ;
#5423=DIRECTION ( 'NONE',  ( 0.000000000000000000, 0.000000000000000000, -1.000000000000000000 ) ) ;
#5426=AXIS2_PLACEMENT_3D ( 'NONE', #7002, #153, #15922 ) ;
#5428=DIRECTION ( 'NONE',  ( 3.469446951953612217E-16, -0.000000000000000000, 1.000000000000000000 ) ) ;
#5429=VERTEX_POINT ( 'NONE', #14409 ) ;
#5434=CIRCLE ( 'NONE', #11960, 10.00000000000000000 ) ;
#5442=ORIENTED_EDGE ( 'NONE', *, *, #1984, .T. ) ;
#5446=DIRECTION ( 'NONE',  ( -1.000000000000000000, 0.000000000000000000, 0.000000000000000000 ) ) ;
#5453=ORIENTED_EDGE ( 'NONE', *, *, #17696, .F. ) ;
#5455=DIRECTION ( 'NONE',  ( -0.000000000000000000, -1.000000000000000000, -0.000000000000000000 ) ) ;
#5460=EDGE_LOOP ( 'NONE', ( #17529, #8611, #14442, #8441 ) ) ;
#5462=VERTEX_POINT ( 'NONE', #11337 ) ;
#5475=VERTEX_POINT ( 'NONE', #15710 ) ;
#5477=ADVANCED_FACE ( 'NONE', ( #1532 ), #7506, .T. ) ;
#5481=DIRECTION ( 'NONE',  ( 1.000000000000000000, 0.000000000000000000, 0.000000000000000000 ) ) ;
#5485=CARTESIAN_POINT ( 'NONE',  ( -1.734723475976807094E-15, 25.39999999999999503, -10.50000000000000178 ) ) ;
#5488=CARTESIAN_POINT ( 'NONE',  ( 9.000000000000001776, 31.99999999999999289, -2.500000000000002665 ) ) ;
#5489=CARTESIAN_POINT ( 'NONE',  ( 8.000000000000000000, 38.59999999999999432, -2.500000000000000888 ) ) ;
#5490=DIRECTION ( 'NONE',  ( 0.000000000000000000, 0.000000000000000000, 1.000000000000000000 ) ) ;
#5491=CARTESIAN_POINT ( 'NONE',  ( -1.734723475976807094E-15, 18.79999999999999361, -2.500000000000000000 ) ) ;
#5497=CARTESIAN_POINT ( 'NONE',  ( 9.999999999999998224, 43.00000000000000000, -2.500000000000001776 ) ) ;
#5501=ADVANCED_FACE ( 'NONE', ( #12912 ), #7803, .T. ) ;
#5505=AXIS2_PLACEMENT_3D ( 'NONE', #12353, #16555, #8184 ) ;
#5508=TOROIDAL_SURFACE ( 'NONE', #4631, 9.000000000000001776, 0.9999999999999991118 ) ;
#5519=FACE_OUTER_BOUND ( 'NONE', #16171, .T. ) ;
#5520=EDGE_CURVE ( 'NONE', #12007, #11229, #16724, .T. ) ;
#5522=CARTESIAN_POINT ( 'NONE',  ( 9.999999999999998224, 38.59999999999999432, -2.500000000000001776 ) ) ;
#5523=CARTESIAN_POINT ( 'NONE',  ( -1.734723475976807094E-15, 23.19999999999999574, -10.50000000000000178 ) ) ;
#5527=CARTESIAN_POINT ( 'NONE',  ( 9.000000000000000000, 16.59999999999999787, -2.500000000000001332 ) ) ;
#5530=ORIENTED_EDGE ( 'NONE', *, *, #4168, .T. ) ;
#5534=CIRCLE ( 'NONE', #6709, 0.9999999999999991118 ) ;
#5536=ORIENTED_EDGE ( 'NONE', *, *, #10577, .F. ) ;
#5540=ORIENTED_EDGE ( 'NONE', *, *, #14255, .T. ) ;
#5542=EDGE_CURVE ( 'NONE', #10845, #13534, #7210, .T. ) ;
#5543=CARTESIAN_POINT ( 'NONE',  ( -1.734723475976807094E-15, 29.79999999999999716, -2.500000000000000000 ) ) ;
#5544=TOROIDAL_SURFACE ( 'NONE', #10878, 9.000000000000003553, 0.9999999999999991118 ) ;
#5553=CARTESIAN_POINT ( 'NONE',  ( 9.999999999999998224, 29.79999999999999716, -2.500000000000001776 ) ) ;
#5560=CIRCLE ( 'NONE', #9391, 0.9999999999999991118 ) ;
#5564=ORIENTED_EDGE ( 'NONE', *, *, #16531, .T. ) ;
#5568=CIRCLE ( 'NONE', #14160, 0.9999999999999991118 ) ;
#5582=ORIENTED_EDGE ( 'NONE', *, *, #11127, .F. ) ;
#5592=STYLED_ITEM('',(#18396),#14621);
#5603=AXIS2_PLACEMENT_3D ( 'NONE', #13135, #4601, #3319 ) ;
#5616=DIRECTION ( 'NONE',  ( -1.000000000000000000, 0.000000000000000000, 4.336808689942021680E-16 ) ) ;
#5620=DIRECTION ( 'NONE',  ( -0.000000000000000000, -1.000000000000000000, -0.000000000000000000 ) ) ;
#5626=CYLINDRICAL_SURFACE ( 'NONE', #1267, 0.9999999999999991118 ) ;
#5628=UNCERTAINTY_MEASURE_WITH_UNIT (LENGTH_MEASURE( 1.000000000000000082E-05 ), #5420, 'distance_accuracy_value', 'NONE');
#5629=CARTESIAN_POINT ( 'NONE',  ( -1.734723475976807094E-15, 40.79999999999999716, -11.50000000000000178 ) ) ;
#5635=VERTEX_POINT ( 'NONE', #2096 ) ;
#5639=DIRECTION ( 'NONE',  ( 0.000000000000000000, 0.000000000000000000, -1.000000000000000000 ) ) ;
#5649=EDGE_CURVE ( 'NONE', #6012, #2199, #7447, .T. ) ;
#5654=ORIENTED_EDGE ( 'NONE', *, *, #17359, .T. ) ;
#5663=DIRECTION ( 'NONE',  ( 0.000000000000000000, 0.000000000000000000, -1.000000000000000000 ) ) ;
#5665=ORIENTED_EDGE ( 'NONE', *, *, #520, .F. ) ;
#5667=FACE_OUTER_BOUND ( 'NONE', #867, .T. ) ;
#5670=( NAMED_UNIT ( * ) PLANE_ANGLE_UNIT ( ) SI_UNIT ( $, .RADIAN. ) );
#5671=ORIENTED_EDGE ( 'NONE', *, *, #11683, .F. ) ;
#5676=AXIS2_PLACEMENT_3D ( 'NONE', #9653, #18037, #13553 ) ;
#5678=DIRECTION ( 'NONE',  ( 3.469446951953612217E-16, -0.000000000000000000, 1.000000000000000000 ) ) ;
#5681=ADVANCED_FACE ( 'NONE', ( #7540 ), #15998, .T. ) ;
#5683=DIRECTION ( 'NONE',  ( -0.000000000000000000, -1.000000000000000000, -0.000000000000000000 ) ) ;
#5688=LINE ( 'NONE', #8828, #11825 ) ;
#5694=DIRECTION ( 'NONE',  ( 1.000000000000000000, 0.000000000000000000, 0.000000000000000000 ) ) ;
#5695=CARTESIAN_POINT ( 'NONE',  ( -8.000000000000001776, 18.79999999999999361, 2.499999999999998224 ) ) ;
#5696=CARTESIAN_POINT ( 'NONE',  ( -1.734723475976807094E-15, 40.79999999999999716, -2.500000000000000000 ) ) ;
#5699=AXIS2_PLACEMENT_3D ( 'NONE', #12027, #10641, #3600 ) ;
#5702=AXIS2_PLACEMENT_3D ( 'NONE', #15946, #17639, #1857 ) ;
#5711=ORIENTED_EDGE ( 'NONE', *, *, #11064, .T. ) ;
#5717=EDGE_LOOP ( 'NONE', ( #17976, #15950, #16496, #11724 ) ) ;
#5721=ORIENTED_EDGE ( 'NONE', *, *, #13575, .T. ) ;
#5724=ADVANCED_FACE ( 'NONE', ( #6433 ), #4256, .T. ) ;
#5725=VERTEX_POINT ( 'NONE', #3475 ) ;
#5729=DIRECTION ( 'NONE',  ( -3.373073425510457965E-16, 0.000000000000000000, -1.000000000000000000 ) ) ;
#5748=AXIS2_PLACEMENT_3D ( 'NONE', #5543, #1112, #5370 ) ;
#5749=DIRECTION ( 'NONE',  ( 0.000000000000000000, 0.000000000000000000, 1.000000000000000000 ) ) ;
#5768=DIRECTION ( 'NONE',  ( 0.000000000000000000, 0.000000000000000000, -1.000000000000000000 ) ) ;
#5776=CARTESIAN_POINT ( 'NONE',  ( -1.734723475976807094E-15, 27.59999999999999432, -11.50000000000000178 ) ) ;
#5779=CARTESIAN_POINT ( 'NONE',  ( -1.734723475976807094E-15, 31.99999999999999289, -2.500000000000000000 ) ) ;
#5781=DIRECTION ( 'NONE',  ( 0.000000000000000000, 0.000000000000000000, -1.000000000000000000 ) ) ;
#5784=ORIENTED_EDGE ( 'NONE', *, *, #7209, .T. ) ;
#5788=DIRECTION ( 'NONE',  ( -1.000000000000000000, 0.000000000000000000, 4.336808689942021680E-16 ) ) ;
#5790=DIRECTION ( 'NONE',  ( -0.000000000000000000, -1.000000000000000000, -0.000000000000000000 ) ) ;
#5804=ADVANCED_FACE ( 'NONE', ( #5039 ), #9301, .T. ) ;
#5811=ORIENTED_EDGE ( 'NONE', *, *, #1747, .T. ) ;
#5821=ORIENTED_EDGE ( 'NONE', *, *, #2645, .T. ) ;
#5830=ORIENTED_EDGE ( 'NONE', *, *, #3989, .F. ) ;
#5832=AXIS2_PLACEMENT_3D ( 'NONE', #3134, #6281, #16129 ) ;
#5834=FACE_OUTER_BOUND ( 'NONE', #7747, .T. ) ;
#5837=DIRECTION ( 'NONE',  ( 0.000000000000000000, 0.000000000000000000, -1.000000000000000000 ) ) ;
#5839=VERTEX_POINT ( 'NONE', #12448 ) ;
#5844=DIRECTION ( 'NONE',  ( -0.000000000000000000, -1.000000000000000000, -0.000000000000000000 ) ) ;
#5852=ADVANCED_FACE ( 'NONE', ( #18141 ), #6023, .T. ) ;
#5859=VECTOR ( 'NONE', #871, 1000.000000000000000 ) ;
#5860=AXIS2_PLACEMENT_3D ( 'NONE', #11510, #7340, #594 ) ;
#5866=DIRECTION ( 'NONE',  ( -0.000000000000000000, -1.000000000000000000, -0.000000000000000000 ) ) ;
#5873=EDGE_CURVE ( 'NONE', #7574, #4547, #10769, .T. ) ;
#5874=AXIS2_PLACEMENT_3D ( 'NONE', #13715, #6848, #5278 ) ;
#5882=CIRCLE ( 'NONE', #12700, 0.9999999999999991118 ) ;
#5893=VECTOR ( 'NONE', #7828, 1000.000000000000000 ) ;
#5900=CARTESIAN_POINT ( 'NONE',  ( -9.000000000000001776, 25.39999999999999503, 2.499999999999998224 ) ) ;
#5909=VERTEX_POINT ( 'NONE', #17949 ) ;
#5911=AXIS2_PLACEMENT_3D ( 'NONE', #14423, #14332, #3299 ) ;
#5913=VERTEX_POINT ( 'NONE', #15156 ) ;
#5921=VERTEX_POINT ( 'NONE', #6698 ) ;
#5924=ORIENTED_EDGE ( 'NONE', *, *, #13749, .T. ) ;
#5932=DIRECTION ( 'NONE',  ( 0.000000000000000000, 0.000000000000000000, 1.000000000000000000 ) ) ;
#5934=ORIENTED_EDGE ( 'NONE', *, *, #10855, .T. ) ;
#5963=ORIENTED_EDGE ( 'NONE', *, *, #12523, .F. ) ;
#5967=ADVANCED_FACE ( 'NONE', ( #16651 ), #12837, .T. ) ;
#5975=LINE ( 'NONE', #13118, #2023 ) ;
#5984=AXIS2_PLACEMENT_3D ( 'NONE', #8875, #12613, #1234 ) ;
#5985=DIRECTION ( 'NONE',  ( 0.000000000000000000, 0.000000000000000000, 1.000000000000000000 ) ) ;
#6002=CARTESIAN_POINT ( 'NONE',  ( 8.000000000000000000, 36.39999999999999147, -2.500000000000000888 ) ) ;
#6003=ORIENTED_EDGE ( 'NONE', *, *, #5062, .F. ) ;
#6004=ORIENTED_EDGE ( 'NONE', *, *, #11127, .T. ) ;
#6012=VERTEX_POINT ( 'NONE', #5497 ) ;
#6016=ORIENTED_EDGE ( 'NONE', *, *, #12317, .F. ) ;
#6023=TOROIDAL_SURFACE ( 'NONE', #14639, 9.000000000000001776, 0.9999999999999991118 ) ;
#6027=CARTESIAN_POINT ( 'NONE',  ( 0.000000000000000000, 38.59999999999999432, 2.500000000000000000 ) ) ;
#6039=ADVANCED_FACE ( 'NONE', ( #14390 ), #4901, .T. ) ;
#6046=DIRECTION ( 'NONE',  ( -1.000000000000000000, 0.000000000000000000, 4.336808689942021680E-16 ) ) ;
#6050=CARTESIAN_POINT ( 'NONE',  ( -10.00000000000000178, 31.99999999999999289, -2.500000000000001776 ) ) ;
#6064=DIRECTION ( 'NONE',  ( -3.469446951953613696E-16, -0.000000000000000000, -1.000000000000000000 ) ) ;
#6080=CIRCLE ( 'NONE', #10226, 0.9999999999999991118 ) ;
#6082=ORIENTED_EDGE ( 'NONE', *, *, #7843, .F. ) ;
#6084=ADVANCED_FACE ( 'NONE', ( #9846 ), #15863, .T. ) ;
#6096=ORIENTED_EDGE ( 'NONE', *, *, #3500, .F. ) ;
#6109=ORIENTED_EDGE ( 'NONE', *, *, #12288, .T. ) ;
#6110=DIRECTION ( 'NONE',  ( 3.469446951953612217E-16, -0.000000000000000000, 1.000000000000000000 ) ) ;
#6115=AXIS2_PLACEMENT_3D ( 'NONE', #8822, #10113, #15797 ) ;
#6124=ORIENTED_EDGE ( 'NONE', *, *, #4555, .F. ) ;
#6138=VECTOR ( 'NONE', #16977, 1000.000000000000000 ) ;
#6140=CARTESIAN_POINT ( 'NONE',  ( 9.000000000000001776, 25.39999999999999503, -2.500000000000002665 ) ) ;
#6148=ORIENTED_EDGE ( 'NONE', *, *, #4955, .F. ) ;
#6159=EDGE_CURVE ( 'NONE', #9378, #6179, #12990, .T. ) ;
#6165=CARTESIAN_POINT ( 'NONE',  ( -1.734723475976807094E-15, 18.79999999999999361, -2.500000000000000000 ) ) ;
#6167=DIRECTION ( 'NONE',  ( 1.000000000000000000, 0.000000000000000000, 0.000000000000000000 ) ) ;
#6168=FACE_OUTER_BOUND ( 'NONE', #8850, .T. ) ;
#6179=VERTEX_POINT ( 'NONE', #15978 ) ;
#6183=AXIS2_PLACEMENT_3D ( 'NONE', #6371, #12015, #2032 ) ;
#6185=CARTESIAN_POINT ( 'NONE',  ( -9.000000000000003553, 38.59999999999999432, -2.500000000000001776 ) ) ;
#6191=ORIENTED_EDGE ( 'NONE', *, *, #14860, .T. ) ;
#6194=DIRECTION ( 'NONE',  ( -0.000000000000000000, -1.000000000000000000, -0.000000000000000000 ) ) ;
#6195=EDGE_LOOP ( 'NONE', ( #6096, #3063, #6109, #16703 ) ) ;
#6196=ORIENTED_EDGE ( 'NONE', *, *, #2416, .T. ) ;
#6198=DIRECTION ( 'NONE',  ( -0.000000000000000000, -1.000000000000000000, -0.000000000000000000 ) ) ;
#6199=VECTOR ( 'NONE', #6909, 1000.000000000000000 ) ;
#6208=CARTESIAN_POINT ( 'NONE',  ( -1.734723475976807094E-15, 36.39999999999999147, -2.500000000000000000 ) ) ;
#6211=CARTESIAN_POINT ( 'NONE',  ( 0.000000000000000000, 25.39999999999999503, 2.500000000000000000 ) ) ;
#6215=FACE_OUTER_BOUND ( 'NONE', #13517, .T. ) ;
#6224=DIRECTION ( 'NONE',  ( -4.915049848600951133E-16, 0.000000000000000000, -1.000000000000000000 ) ) ;
#6237=CARTESIAN_POINT ( 'NONE',  ( -10.00000000000000000, 20.99999999999999289, 2.499999999999998224 ) ) ;
#6241=EDGE_LOOP ( 'NONE', ( #16116, #18034, #8046, #10355 ) ) ;
#6249=EDGE_CURVE ( 'NONE', #5913, #12253, #16465, .T. ) ;
#6250=CIRCLE ( 'NONE', #6550, 10.00000000000000178 ) ;
#6258=EDGE_LOOP ( 'NONE', ( #12529, #18105, #15415, #912 ) ) ;
#6259=DIRECTION ( 'NONE',  ( -0.000000000000000000, -1.000000000000000000, -0.000000000000000000 ) ) ;
#6260=DIRECTION ( 'NONE',  ( 0.000000000000000000, 0.000000000000000000, -1.000000000000000000 ) ) ;
#6262=ORIENTED_EDGE ( 'NONE', *, *, #4316, .F. ) ;
#6268=ADVANCED_FACE ( 'NONE', ( #16732 ), #1239, .T. ) ;
#6269=ORIENTED_EDGE ( 'NONE', *, *, #4387, .F. ) ;
#6278=CIRCLE ( 'NONE', #11601, 0.9999999999999991118 ) ;
#6281=DIRECTION ( 'NONE',  ( -0.000000000000000000, -1.000000000000000000, -0.000000000000000000 ) ) ;
#6285=CIRCLE ( 'NONE', #7762, 0.9999999999999991118 ) ;
#6287=AXIS2_PLACEMENT_3D ( 'NONE', #13075, #3263, #669 ) ;
#6289=ORIENTED_EDGE ( 'NONE', *, *, #14069, .T. ) ;
#6292=( NAMED_UNIT ( * ) SI_UNIT ( $, .STERADIAN. ) SOLID_ANGLE_UNIT ( ) );
#6302=CIRCLE ( 'NONE', #14279, 0.9999999999999991118 ) ;
#6313=CARTESIAN_POINT ( 'NONE',  ( 10.00000000000000355, 34.19999999999999574, 2.499999999999996891 ) ) ;
#6314=CIRCLE ( 'NONE', #1280, 0.9999999999999991118 ) ;
#6317=ORIENTED_EDGE ( 'NONE', *, *, #16020, .F. ) ;
#6318=CIRCLE ( 'NONE', #3644, 10.00000000000000000 ) ;
#6323=EDGE_CURVE ( 'NONE', #12786, #2131, #14704, .T. ) ;
#6327=EDGE_CURVE ( 'NONE', #9609, #1200, #2561, .T. ) ;
#6332=DIRECTION ( 'NONE',  ( -0.000000000000000000, -1.000000000000000000, -0.000000000000000000 ) ) ;
#6338=DIRECTION ( 'NONE',  ( 0.000000000000000000, 0.000000000000000000, 1.000000000000000000 ) ) ;
#6347=DIRECTION ( 'NONE',  ( -0.000000000000000000, -1.000000000000000000, -0.000000000000000000 ) ) ;
#6353=DIRECTION ( 'NONE',  ( 0.000000000000000000, 0.000000000000000000, 1.000000000000000000 ) ) ;
#6355=STYLED_ITEM('',(#18396),#8351);
#6365=DIRECTION ( 'NONE',  ( 0.000000000000000000, 0.000000000000000000, -1.000000000000000000 ) ) ;
#6366=VERTEX_POINT ( 'NONE', #5489 ) ;
#6371=CARTESIAN_POINT ( 'NONE',  ( 0.000000000000000000, 18.79999999999999361, 2.500000000000000000 ) ) ;
#6377=ADVANCED_FACE ( 'NONE', ( #16 ), #8439, .T. ) ;
#6385=( NAMED_UNIT ( * ) SI_UNIT ( $, .STERADIAN. ) SOLID_ANGLE_UNIT ( ) );
#6394=EDGE_LOOP ( 'NONE', ( #15128, #473, #13236, #6661 ) ) ;
#6426=ORIENTED_EDGE ( 'NONE', *, *, #1184, .T. ) ;
#6428=DIRECTION ( 'NONE',  ( 1.000000000000000000, 0.000000000000000000, 0.000000000000000000 ) ) ;
#6429=CIRCLE ( 'NONE', #10262, 10.00000000000000000 ) ;
#6432=ADVANCED_FACE ( 'NONE', ( #976 ), #15437, .T. ) ;
#6433=FACE_OUTER_BOUND ( 'NONE', #2336, .T. ) ;
#6437=TOROIDAL_SURFACE ( 'NONE', #14436, 9.000000000000001776, 0.9999999999999991118 ) ;
#6440=CARTESIAN_POINT ( 'NONE',  ( 9.000000000000001776, 36.39999999999999147, -2.500000000000002665 ) ) ;
#6442=ORIENTED_EDGE ( 'NONE', *, *, #13039, .T. ) ;
#6447=ORIENTED_EDGE ( 'NONE', *, *, #15347, .T. ) ;
#6459=CIRCLE ( 'NONE', #15636, 10.00000000000000000 ) ;
#6468=ORIENTED_EDGE ( 'NONE', *, *, #10633, .T. ) ;
#6477=EDGE_LOOP ( 'NONE', ( #15112, #7532, #533, #13690 ) ) ;
#6480=ADVANCED_FACE ( 'NONE', ( #8092 ), #8454, .T. ) ;
#6490=ORIENTED_EDGE ( 'NONE', *, *, #3723, .T. ) ;
#6504=ORIENTED_EDGE ( 'NONE', *, *, #16945, .F. ) ;
#6507=STYLED_ITEM('',(#18396),#7672);
#6509=DIRECTION ( 'NONE',  ( 0.000000000000000000, 0.000000000000000000, -1.000000000000000000 ) ) ;
#6511=AXIS2_PLACEMENT_3D ( 'NONE', #8920, #5031, #10686 ) ;
#6512=DIRECTION ( 'NONE',  ( 0.000000000000000000, 0.000000000000000000, -1.000000000000000000 ) ) ;
#6515=DIRECTION ( 'NONE',  ( 3.469446951953612217E-16, -0.000000000000000000, 1.000000000000000000 ) ) ;
#6518=ORIENTED_EDGE ( 'NONE', *, *, #9660, .F. ) ;
#6522=DIRECTION ( 'NONE',  ( -0.000000000000000000, -1.000000000000000000, -0.000000000000000000 ) ) ;
#6529=DIRECTION ( 'NONE',  ( -1.000000000000000000, 0.000000000000000000, 0.000000000000000000 ) ) ;
#6532=FACE_OUTER_BOUND ( 'NONE', #17800, .T. ) ;
#6544=ORIENTED_EDGE ( 'NONE', *, *, #11117, .F. ) ;
#6545=ADVANCED_FACE ( 'NONE', ( #15257 ), #16835, .T. ) ;
#6550=AXIS2_PLACEMENT_3D ( 'NONE', #3397, #891, #13483 ) ;
#6552=EDGE_CURVE ( 'NONE', #17766, #3719, #14095, .T. ) ;
#6555=EDGE_LOOP ( 'NONE', ( #10273, #2787, #3013, #2135 ) ) ;
#6556=FACE_OUTER_BOUND ( 'NONE', #9251, .T. ) ;
#6569=ORIENTED_EDGE ( 'NONE', *, *, #5294, .T. ) ;
#6578=ORIENTED_EDGE ( 'NONE', *, *, #7259, .T. ) ;
#6580=AXIS2_PLACEMENT_3D ( 'NONE', #6772, #8348, #2443 ) ;
#6595=ORIENTED_EDGE ( 'NONE', *, *, #9977, .T. ) ;
#6598=DIRECTION ( 'NONE',  ( 0.000000000000000000, 0.000000000000000000, -1.000000000000000000 ) ) ;
#6601=CIRCLE ( 'NONE', #4519, 0.9999999999999991118 ) ;
#6609=ADVANCED_FACE ( 'NONE', ( #15157 ), #12012, .T. ) ;
#6610=ADVANCED_FACE ( 'NONE', ( #16742 ), #18318, .T. ) ;
#6611=CARTESIAN_POINT ( 'NONE',  ( -1.734723475976807094E-15, 16.59999999999999787, -2.500000000000000000 ) ) ;
#6613=VERTEX_POINT ( 'NONE', #8282 ) ;
#6630=CARTESIAN_POINT ( 'NONE',  ( -9.000000000000001776, 38.59999999999999432, 2.499999999999998224 ) ) ;
#6636=ORIENTED_EDGE ( 'NONE', *, *, #15742, .F. ) ;
#6638=EDGE_CURVE ( 'NONE', #11926, #12347, #4199, .T. ) ;
#6645=VERTEX_POINT ( 'NONE', #9847 ) ;
#6646=DIRECTION ( 'NONE',  ( -4.915049848600951133E-16, 0.000000000000000000, -1.000000000000000000 ) ) ;
#6650=ORIENTED_EDGE ( 'NONE', *, *, #4551, .F. ) ;
#6661=ORIENTED_EDGE ( 'NONE', *, *, #17545, .T. ) ;
#6667=CARTESIAN_POINT ( 'NONE',  ( 9.000000000000005329, 29.79999999999999716, 2.499999999999997335 ) ) ;
#6670=DIRECTION ( 'NONE',  ( -3.469446951953613696E-16, -0.000000000000000000, -1.000000000000000000 ) ) ;
#6680=EDGE_LOOP ( 'NONE', ( #8978, #1993, #1506, #4040 ) ) ;
#6686=CYLINDRICAL_SURFACE ( 'NONE', #5042, 0.9999999999999991118 ) ;
#6689=DIRECTION ( 'NONE',  ( 0.000000000000000000, 0.000000000000000000, -1.000000000000000000 ) ) ;
#6698=CARTESIAN_POINT ( 'NONE',  ( -10.00000000000000178, 40.79999999999999716, -2.500000000000001776 ) ) ;
#6701=EDGE_CURVE ( 'NONE', #2806, #9378, #13794, .T. ) ;
#6704=CARTESIAN_POINT ( 'NONE',  ( -1.734723475976807094E-15, 43.00000000000000000, -2.500000000000000000 ) ) ;
#6707=FACE_OUTER_BOUND ( 'NONE', #7650, .T. ) ;
#6709=AXIS2_PLACEMENT_3D ( 'NONE', #772, #2356, #9375 ) ;
#6718=DIRECTION ( 'NONE',  ( -0.000000000000000000, -1.000000000000000000, -0.000000000000000000 ) ) ;
#6719=ADVANCED_FACE ( 'NONE', ( #10109 ), #11322, .T. ) ;
#6730=DIRECTION ( 'NONE',  ( -1.000000000000000000, 0.000000000000000000, 0.000000000000000000 ) ) ;
#6735=AXIS2_PLACEMENT_3D ( 'NONE', #3424, #9400, #2474 ) ;
#6739=FACE_OUTER_BOUND ( 'NONE', #11852, .T. ) ;
#6750=AXIS2_PLACEMENT_3D ( 'NONE', #11221, #14195, #1498 ) ;
#6768=ORIENTED_EDGE ( 'NONE', *, *, #5542, .T. ) ;
#6772=CARTESIAN_POINT ( 'NONE',  ( -9.000000000000001776, 27.59999999999999432, 2.499999999999995559 ) ) ;
#6778=EDGE_CURVE ( 'NONE', #2439, #8594, #12174, .T. ) ;
#6779=DIRECTION ( 'NONE',  ( -0.000000000000000000, -1.000000000000000000, -0.000000000000000000 ) ) ;
#6780=EDGE_LOOP ( 'NONE', ( #17606, #3611, #189, #9160 ) ) ;
#6783=DIRECTION ( 'NONE',  ( 0.000000000000000000, 0.000000000000000000, -1.000000000000000000 ) ) ;
#6784=CIRCLE ( 'NONE', #10637, 0.9999999999999991118 ) ;
#6785=FACE_OUTER_BOUND ( 'NONE', #11797, .T. ) ;
#6800=DIRECTION ( 'NONE',  ( -3.469446951953613696E-16, -0.000000000000000000, -1.000000000000000000 ) ) ;
#6801=AXIS2_PLACEMENT_3D ( 'NONE', #13853, #15442, #4021 ) ;
#6803=FACE_OUTER_BOUND ( 'NONE', #4150, .T. ) ;
#6808=DIRECTION ( 'NONE',  ( -3.469446951953613696E-16, -0.000000000000000000, -1.000000000000000000 ) ) ;
#6810=CARTESIAN_POINT ( 'NONE',  ( 9.000000000000001776, 34.19999999999999574, -2.500000000000002665 ) ) ;
#6813=DIRECTION ( 'NONE',  ( -0.000000000000000000, -1.000000000000000000, -0.000000000000000000 ) ) ;
#6822=DIRECTION ( 'NONE',  ( -1.000000000000000000, 0.000000000000000000, 4.336808689942021680E-16 ) ) ;
#6827=AXIS2_PLACEMENT_3D ( 'NONE', #5164, #10818, #16493 ) ;
#6834=EDGE_CURVE ( 'NONE', #15647, #8512, #17133, .T. ) ;
#6844=DIRECTION ( 'NONE',  ( -1.000000000000000000, 0.000000000000000000, 4.336808689942021680E-16 ) ) ;
#6848=DIRECTION ( 'NONE',  ( -1.000000000000000000, 0.000000000000000000, 0.000000000000000000 ) ) ;
#6851=CARTESIAN_POINT ( 'NONE',  ( 9.000000000000000000, 20.99999999999999289, -2.500000000000001332 ) ) ;
#6852=CARTESIAN_POINT ( 'NONE',  ( 9.000000000000005329, 31.99999999999999289, 2.499999999999997335 ) ) ;
#6854=VERTEX_POINT ( 'NONE', #15504 ) ;
#6862=AXIS2_PLACEMENT_3D ( 'NONE', #8595, #8780, #12956 ) ;
#6871=DIRECTION ( 'NONE',  ( -3.469446951953613696E-16, -0.000000000000000000, -1.000000000000000000 ) ) ;
#6873=AXIS2_PLACEMENT_3D ( 'NONE', #17329, #17420, #10619 ) ;
#6876=TOROIDAL_SURFACE ( 'NONE', #13694, 9.000000000000003553, 0.9999999999999991118 ) ;
#6880=EDGE_CURVE ( 'NONE', #6012, #5909, #13849, .T. ) ;
#6883=DIRECTION ( 'NONE',  ( 0.000000000000000000, 0.000000000000000000, -1.000000000000000000 ) ) ;
#6885=CIRCLE ( 'NONE', #17280, 8.000000000000001776 ) ;
#6889=CARTESIAN_POINT ( 'NONE',  ( -1.734723475976807094E-15, 40.79999999999999716, -2.500000000000000000 ) ) ;
#6890=DIRECTION ( 'NONE',  ( 0.000000000000000000, 0.000000000000000000, -1.000000000000000000 ) ) ;
#6897=CARTESIAN_POINT ( 'NONE',  ( -1.734723475976807094E-15, 34.19999999999999574, -2.500000000000000000 ) ) ;
#6898=AXIS2_PLACEMENT_3D ( 'NONE', #12371, #5428, #9500 ) ;
#6899=CIRCLE ( 'NONE', #11620, 8.000000000000001776 ) ;
#6901=EDGE_CURVE ( 'NONE', #17767, #6613, #4090, .T. ) ;
#6905=DIRECTION ( 'NONE',  ( -3.373073425510457965E-16, 0.000000000000000000, -1.000000000000000000 ) ) ;
#6907=CYLINDRICAL_SURFACE ( 'NONE', #14405, 0.9999999999999991118 ) ;
#6908=AXIS2_PLACEMENT_3D ( 'NONE', #7817, #3388, #11802 ) ;
#6909=DIRECTION ( 'NONE',  ( -3.469446951953613696E-16, -0.000000000000000000, -1.000000000000000000 ) ) ;
#6912=ORIENTED_EDGE ( 'NONE', *, *, #7203, .F. ) ;
#6927=( LENGTH_UNIT ( ) NAMED_UNIT ( * ) SI_UNIT ( .MILLI., .METRE. ) );
#6939=DIRECTION ( 'NONE',  ( -0.000000000000000000, -1.000000000000000000, -0.000000000000000000 ) ) ;
#6977=DIRECTION ( 'NONE',  ( -0.000000000000000000, -1.000000000000000000, -0.000000000000000000 ) ) ;
#6996=CARTESIAN_POINT ( 'NONE',  ( -1.734723475976807094E-15, 20.99999999999999289, -12.50000000000000000 ) ) ;
#7002=CARTESIAN_POINT ( 'NONE',  ( -9.000000000000003553, 34.19999999999999574, -2.500000000000001776 ) ) ;
#7003=TOROIDAL_SURFACE ( 'NONE', #2868, 9.000000000000003553, 0.9999999999999991118 ) ;
#7011=AXIS2_PLACEMENT_3D ( 'NONE', #1165, #8104, #10799 ) ;
#7017=ORIENTED_EDGE ( 'NONE', *, *, #16695, .T. ) ;
#7021=CARTESIAN_POINT ( 'NONE',  ( 0.000000000000000000, 16.59999999999999787, 2.500000000000000000 ) ) ;
#7024=AXIS2_PLACEMENT_3D ( 'NONE', #18060, #13668, #3849 ) ;
#7028=EDGE_CURVE ( 'NONE', #9017, #18266, #2627, .T. ) ;
#7032=AXIS2_PLACEMENT_3D ( 'NONE', #5045, #3842, #2106 ) ;
#7041=AXIS2_PLACEMENT_3D ( 'NONE', #13834, #6871, #16731 ) ;
#7043=ORIENTED_EDGE ( 'NONE', *, *, #137, .T. ) ;
#7044=CIRCLE ( 'NONE', #5860, 8.000000000000001776 ) ;
#7045=VERTEX_POINT ( 'NONE', #8514 ) ;
#7048=DIRECTION ( 'NONE',  ( 0.000000000000000000, 0.000000000000000000, -1.000000000000000000 ) ) ;
#7064=CARTESIAN_POINT ( 'NONE',  ( -1.734723475976807094E-15, 29.79999999999999716, -2.500000000000000000 ) ) ;
#7066=CYLINDRICAL_SURFACE ( 'NONE', #16281, 0.9999999999999991118 ) ;
#7069=AXIS2_PLACEMENT_3D ( 'NONE', #12467, #4134, #9604 ) ;
#7080=CIRCLE ( 'NONE', #11516, 0.9999999999999991118 ) ;
#7081=DIRECTION ( 'NONE',  ( -0.000000000000000000, -1.000000000000000000, -0.000000000000000000 ) ) ;
#7082=CIRCLE ( 'NONE', #16599, 10.00000000000000178 ) ;
#7084=DIRECTION ( 'NONE',  ( -1.000000000000000000, 0.000000000000000000, 4.336808689942021680E-16 ) ) ;
#7088=EDGE_LOOP ( 'NONE', ( #4527, #363, #12393, #10832 ) ) ;
#7092=ORIENTED_EDGE ( 'NONE', *, *, #4316, .T. ) ;
#7093=DIRECTION ( 'NONE',  ( 0.000000000000000000, 0.000000000000000000, 1.000000000000000000 ) ) ;
#7096=AXIS2_PLACEMENT_3D ( 'NONE', #6889, #18148, #13661 ) ;
#7103=EDGE_CURVE ( 'NONE', #17729, #17010, #1168, .T. ) ;
#7106=EDGE_CURVE ( 'NONE', #11668, #4985, #14481, .T. ) ;
#7107=DIRECTION ( 'NONE',  ( -4.915049848600951133E-16, 0.000000000000000000, -1.000000000000000000 ) ) ;
#7109=VECTOR ( 'NONE', #17020, 1000.000000000000000 ) ;
#7113=ORIENTED_EDGE ( 'NONE', *, *, #141, .F. ) ;
#7116=ORIENTED_EDGE ( 'NONE', *, *, #8542, .T. ) ;
#7126=AXIS2_PLACEMENT_3D ( 'NONE', #9866, #10041, #8467 ) ;
#7134=VERTEX_POINT ( 'NONE', #13522 ) ;
#7139=DIRECTION ( 'NONE',  ( 0.000000000000000000, 0.000000000000000000, -1.000000000000000000 ) ) ;
#7152=EDGE_CURVE ( 'NONE', #17369, #634, #2372, .T. ) ;
#7153=AXIS2_PLACEMENT_3D ( 'NONE', #10286, #4277, #17277 ) ;
#7155=AXIS2_PLACEMENT_3D ( 'NONE', #10481, #579, #1786 ) ;
#7157=CARTESIAN_POINT ( 'NONE',  ( -8.000000000000001776, 43.00000000000000000, 2.499999999999998224 ) ) ;
#7165=DIRECTION ( 'NONE',  ( 0.000000000000000000, 0.000000000000000000, 1.000000000000000000 ) ) ;
#7176=DIRECTION ( 'NONE',  ( -0.000000000000000000, -1.000000000000000000, -0.000000000000000000 ) ) ;
#7178=CARTESIAN_POINT ( 'NONE',  ( 8.000000000000000000, 25.39999999999999503, -2.500000000000000888 ) ) ;
#7182=CIRCLE ( 'NONE', #1578, 8.000000000000003553 ) ;
#7188=CARTESIAN_POINT ( 'NONE',  ( 9.000000000000000000, 25.39999999999999503, -2.500000000000001332 ) ) ;
#7189=EDGE_CURVE ( 'NONE', #9963, #9627, #17779, .T. ) ;
#7192=ORIENTED_EDGE ( 'NONE', *, *, #15238, .F. ) ;
#7196=AXIS2_PLACEMENT_3D ( 'NONE', #12462, #6718, #13581 ) ;
#7203=EDGE_CURVE ( 'NONE', #5462, #17357, #2948, .T. ) ;
#7205=DIRECTION ( 'NONE',  ( -1.000000000000000000, 0.000000000000000000, 4.336808689942021680E-16 ) ) ;
#7207=EDGE_LOOP ( 'NONE', ( #3004, #5811, #9918, #15639 ) ) ;
#7209=EDGE_CURVE ( 'NONE', #12253, #15689, #17179, .T. ) ;
#7210=CIRCLE ( 'NONE', #6908, 8.000000000000001776 ) ;
#7218=ORIENTED_EDGE ( 'NONE', *, *, #13174, .T. ) ;
#7224=ADVANCED_FACE ( 'NONE', ( #14568 ), #1768, .T. ) ;
#7228=DIRECTION ( 'NONE',  ( -0.000000000000000000, -1.000000000000000000, -0.000000000000000000 ) ) ;
#7233=DIRECTION ( 'NONE',  ( -0.000000000000000000, -1.000000000000000000, -0.000000000000000000 ) ) ;
#7244=CARTESIAN_POINT ( 'NONE',  ( 8.000000000000000000, 20.99999999999999289, -2.500000000000000888 ) ) ;
#7259=EDGE_CURVE ( 'NONE', #9627, #4165, #467, .T. ) ;
#7261=DIRECTION ( 'NONE',  ( -4.915049848600951133E-16, 0.000000000000000000, -1.000000000000000000 ) ) ;
#7267=CARTESIAN_POINT ( 'NONE',  ( -9.000000000000001776, 27.59999999999999432, 2.499999999999998224 ) ) ;
#7273=EDGE_LOOP ( 'NONE', ( #6082, #15993, #4567, #17659 ) ) ;
#7278=DIRECTION ( 'NONE',  ( -0.000000000000000000, -1.000000000000000000, -0.000000000000000000 ) ) ;
#7283=TOROIDAL_SURFACE ( 'NONE', #12628, 9.000000000000001776, 0.9999999999999991118 ) ;
#7295=CIRCLE ( 'NONE', #17706, 10.00000000000000178 ) ;
#7298=CARTESIAN_POINT ( 'NONE',  ( -9.000000000000001776, 23.19999999999999574, 2.499999999999998224 ) ) ;
#7307=CARTESIAN_POINT ( 'NONE',  ( -9.000000000000001776, 34.19999999999999574, 2.499999999999998224 ) ) ;
#7308=CIRCLE ( 'NONE', #12349, 8.000000000000001776 ) ;
#7313=DIRECTION ( 'NONE',  ( -1.000000000000000000, 0.000000000000000000, 0.000000000000000000 ) ) ;
#7324=CIRCLE ( 'NONE', #7032, 0.9999999999999991118 ) ;
#7333=AXIS2_PLACEMENT_3D ( 'NONE', #5779, #4481, #17112 ) ;
#7334=ADVANCED_FACE ( 'NONE', ( #3972 ), #3833, .T. ) ;
#7336=MECHANICAL_DESIGN_GEOMETRIC_PRESENTATION_REPRESENTATION('',(#17434),#9707);
#7340=DIRECTION ( 'NONE',  ( -0.000000000000000000, -1.000000000000000000, -0.000000000000000000 ) ) ;
#7344=ORIENTED_EDGE ( 'NONE', *, *, #12378, .F. ) ;
#7349=AXIS2_PLACEMENT_3D ( 'NONE', #2329, #7958, #3789 ) ;
#7371=DIRECTION ( 'NONE',  ( 0.000000000000000000, 0.000000000000000000, 1.000000000000000000 ) ) ;
#7375=AXIS2_PLACEMENT_3D ( 'NONE', #8238, #1209, #14167 ) ;
#7385=EDGE_CURVE ( 'NONE', #4165, #17338, #9166, .T. ) ;
#7389=CIRCLE ( 'NONE', #7995, 8.000000000000001776 ) ;
#7390=LINE ( 'NONE', #8776, #9975 ) ;
#7394=DIRECTION ( 'NONE',  ( -1.000000000000000000, 0.000000000000000000, 4.336808689942021680E-16 ) ) ;
#7395=CARTESIAN_POINT ( 'NONE',  ( -9.000000000000001776, 16.59999999999999787, 2.499999999999998224 ) ) ;
#7400=ORIENTED_EDGE ( 'NONE', *, *, #15392, .F. ) ;
#7404=AXIS2_PLACEMENT_3D ( 'NONE', #13738, #2447, #3910 ) ;
#7414=DIRECTION ( 'NONE',  ( 0.000000000000000000, 0.000000000000000000, -1.000000000000000000 ) ) ;
#7415=CARTESIAN_POINT ( 'NONE',  ( -1.734723475976807094E-15, 38.59999999999999432, -2.500000000000000000 ) ) ;
#7430=CARTESIAN_POINT ( 'NONE',  ( 8.000000000000000000, 18.79999999999999361, -2.500000000000000888 ) ) ;
#7440=ORIENTED_EDGE ( 'NONE', *, *, #16027, .T. ) ;
#7441=TOROIDAL_SURFACE ( 'NONE', #8345, 9.000000000000001776, 0.9999999999999991118 ) ;
#7447=LINE ( 'NONE', #3291, #4545 ) ;
#7453=CARTESIAN_POINT ( 'NONE',  ( -1.734723475976807094E-15, 20.99999999999999289, -2.500000000000000000 ) ) ;
#7456=CARTESIAN_POINT ( 'NONE',  ( 9.000000000000005329, 25.39999999999999503, 2.499999999999997335 ) ) ;
#7460=DIRECTION ( 'NONE',  ( -4.915049848600951133E-16, 0.000000000000000000, -1.000000000000000000 ) ) ;
#7478=CIRCLE ( 'NONE', #11932, 10.00000000000000000 ) ;
#7479=DIRECTION ( 'NONE',  ( -0.000000000000000000, -1.000000000000000000, -0.000000000000000000 ) ) ;
#7480=CIRCLE ( 'NONE', #1282, 10.00000000000000000 ) ;
#7483=EDGE_LOOP ( 'NONE', ( #4599, #8010, #14111, #14680 ) ) ;
#7486=CARTESIAN_POINT ( 'NONE',  ( -10.00000000000000000, 31.99999999999999289, 2.499999999999998224 ) ) ;
#7487=ORIENTED_EDGE ( 'NONE', *, *, #2747, .T. ) ;
#7499=DIRECTION ( 'NONE',  ( 0.000000000000000000, 0.000000000000000000, -1.000000000000000000 ) ) ;
#7506=TOROIDAL_SURFACE ( 'NONE', #2505, 9.000000000000001776, 0.9999999999999991118 ) ;
#7508=EDGE_CURVE ( 'NONE', #2199, #11229, #7082, .T. ) ;
#7510=ORIENTED_EDGE ( 'NONE', *, *, #131, .F. ) ;
#7528=CARTESIAN_POINT ( 'NONE',  ( 0.000000000000000000, 31.99999999999999289, 2.500000000000000000 ) ) ;
#7530=DIRECTION ( 'NONE',  ( -4.915049848600951133E-16, 0.000000000000000000, -1.000000000000000000 ) ) ;
#7531=ORIENTED_EDGE ( 'NONE', *, *, #14532, .T. ) ;
#7532=ORIENTED_EDGE ( 'NONE', *, *, #17898, .T. ) ;
#7534=CARTESIAN_POINT ( 'NONE',  ( 9.000000000000001776, 43.00000000000000000, -2.500000000000002665 ) ) ;
#7540=FACE_OUTER_BOUND ( 'NONE', #10210, .T. ) ;
#7551=CARTESIAN_POINT ( 'NONE',  ( -8.000000000000001776, 34.19999999999999574, 2.499999999999995115 ) ) ;
#7552=CARTESIAN_POINT ( 'NONE',  ( 9.000000000000001776, 27.59999999999999432, -2.500000000000002665 ) ) ;
#7564=AXIS2_PLACEMENT_3D ( 'NONE', #11136, #1418, #14107 ) ;
#7567=CARTESIAN_POINT ( 'NONE',  ( 0.000000000000000000, 40.79999999999999716, 2.500000000000000000 ) ) ;
#7574=VERTEX_POINT ( 'NONE', #2950 ) ;
#7575=CARTESIAN_POINT ( 'NONE',  ( -1.734723475976807094E-15, 34.19999999999999574, -2.500000000000000000 ) ) ;
#7594=AXIS2_PLACEMENT_3D ( 'NONE', #17669, #6332, #863 ) ;
#7602=ORIENTED_EDGE ( 'NONE', *, *, #1845, .T. ) ;
#7616=CYLINDRICAL_SURFACE ( 'NONE', #4979, 0.9999999999999991118 ) ;
#7621=DIRECTION ( 'NONE',  ( -1.000000000000000000, 0.000000000000000000, 0.000000000000000000 ) ) ;
#7623=ORIENTED_EDGE ( 'NONE', *, *, #3500, .T. ) ;
#7630=DIRECTION ( 'NONE',  ( -0.000000000000000000, -1.000000000000000000, -0.000000000000000000 ) ) ;
#7644=CIRCLE ( 'NONE', #14483, 8.000000000000003553 ) ;
#7650=EDGE_LOOP ( 'NONE', ( #719, #1368, #4733, #12066 ) ) ;
#7668=EDGE_LOOP ( 'NONE', ( #3776, #7892, #9968, #15739 ) ) ;
#7669=ORIENTED_EDGE ( 'NONE', *, *, #844, .F. ) ;
#7672=MANIFOLD_SOLID_BREP ( 'Sweep1', #7922 ) ;
#7673=CARTESIAN_POINT ( 'NONE',  ( 0.000000000000000000, 20.99999999999999289, 2.500000000000000000 ) ) ;
#7679=EDGE_CURVE ( 'NONE', #894, #3649, #15119, .T. ) ;
#7684=SHAPE_REPRESENTATION ( 'coil', ( #16940 ), #11010 ) ;
#7703=AXIS2_PLACEMENT_3D ( 'NONE', #3373, #14595, #2082 ) ;
#7707=MANIFOLD_SOLID_BREP ( 'LPattern6[2]', #15343 ) ;
#7713=DIRECTION ( 'NONE',  ( -0.000000000000000000, -1.000000000000000000, -0.000000000000000000 ) ) ;
#7714=DIRECTION ( 'NONE',  ( 0.000000000000000000, 0.000000000000000000, 1.000000000000000000 ) ) ;
#7723=CARTESIAN_POINT ( 'NONE',  ( 0.000000000000000000, 20.99999999999999289, 2.500000000000000000 ) ) ;
#7731=DIRECTION ( 'NONE',  ( 1.000000000000000000, 0.000000000000000000, 0.000000000000000000 ) ) ;
#7732=ADVANCED_FACE ( 'NONE', ( #11735 ), #15464, .T. ) ;
#7740=ADVANCED_FACE ( 'NONE', ( #9240 ), #1941, .T. ) ;
#7747=EDGE_LOOP ( 'NONE', ( #8987, #2085, #4461, #1854 ) ) ;
#7751=ORIENTED_EDGE ( 'NONE', *, *, #13676, .F. ) ;
#7753=( NAMED_UNIT ( * ) PLANE_ANGLE_UNIT ( ) SI_UNIT ( $, .RADIAN. ) );
#7760=ORIENTED_EDGE ( 'NONE', *, *, #4955, .T. ) ;
#7762=AXIS2_PLACEMENT_3D ( 'NONE', #8574, #7093, #345 ) ;
#7767=DIRECTION ( 'NONE',  ( -1.000000000000000000, 0.000000000000000000, 4.336808689942021680E-16 ) ) ;
#7768=FILL_AREA_STYLE ('',( #10547 ) ) ;
#7775=EDGE_LOOP ( 'NONE', ( #13991, #4317, #15928, #5267 ) ) ;
#7776=AXIS2_PLACEMENT_3D ( 'NONE', #3543, #12143, #764 ) ;
#7803=TOROIDAL_SURFACE ( 'NONE', #3966, 9.000000000000001776, 0.9999999999999991118 ) ;
#7809=ORIENTED_EDGE ( 'NONE', *, *, #14860, .F. ) ;
#7817=CARTESIAN_POINT ( 'NONE',  ( -1.734723475976807094E-15, 38.59999999999999432, -2.500000000000000000 ) ) ;
#7818=FACE_OUTER_BOUND ( 'NONE', #9145, .T. ) ;
#7822=MANIFOLD_SOLID_BREP ( 'LPattern6[1]', #11169 ) ;
#7828=DIRECTION ( 'NONE',  ( -3.469446951953613696E-16, -0.000000000000000000, -1.000000000000000000 ) ) ;
#7840=ADVANCED_FACE ( 'NONE', ( #16671 ), #4264, .T. ) ;
#7843=EDGE_CURVE ( 'NONE', #3136, #7134, #10786, .T. ) ;
#7844=CARTESIAN_POINT ( 'NONE',  ( 9.000000000000005329, 27.59999999999999432, 2.499999999999997335 ) ) ;
#7845=CARTESIAN_POINT ( 'NONE',  ( -9.000000000000001776, 20.99999999999999289, 2.499999999999995559 ) ) ;
#7851=DIRECTION ( 'NONE',  ( -3.373073425510457965E-16, 0.000000000000000000, -1.000000000000000000 ) ) ;
#7859=AXIS2_PLACEMENT_3D ( 'NONE', #2819, #12723, #5768 ) ;
#7884=ORIENTED_EDGE ( 'NONE', *, *, #8063, .F. ) ;
#7886=VECTOR ( 'NONE', #12108, 1000.000000000000000 ) ;
#7892=ORIENTED_EDGE ( 'NONE', *, *, #10176, .T. ) ;
#7909=AXIS2_PLACEMENT_3D ( 'NONE', #6630, #2041, #8013 ) ;
#7910=AXIS2_PLACEMENT_3D ( 'NONE', #8496, #12433, #17151 ) ;
#7916=ORIENTED_EDGE ( 'NONE', *, *, #4453, .F. ) ;
#7918=LINE ( 'NONE', #10704, #15396 ) ;
#7920=ORIENTED_EDGE ( 'NONE', *, *, #12163, .T. ) ;
#7922=CLOSED_SHELL ( 'NONE', ( #17569, #2488, #10265, #16458, #945, #3506, #16836, #8167, #12633, #10624 ) ) ;
#7925=VECTOR ( 'NONE', #3051, 1000.000000000000000 ) ;
#7928=ORIENTED_EDGE ( 'NONE', *, *, #16926, .T. ) ;
#7933=EDGE_CURVE ( 'NONE', #4719, #3449, #6080, .T. ) ;
#7934=CARTESIAN_POINT ( 'NONE',  ( 0.000000000000000000, 16.59999999999999787, 2.500000000000000000 ) ) ;
#7937=AXIS2_PLACEMENT_3D ( 'NONE', #2358, #13643, #960 ) ;
#7941=ORIENTED_EDGE ( 'NONE', *, *, #11537, .T. ) ;
#7958=DIRECTION ( 'NONE',  ( 0.000000000000000000, 0.000000000000000000, 1.000000000000000000 ) ) ;
#7959=EDGE_CURVE ( 'NONE', #14652, #17766, #17885, .T. ) ;
#7963=EDGE_CURVE ( 'NONE', #5212, #12374, #8759, .T. ) ;
#7966=CIRCLE ( 'NONE', #10327, 10.00000000000000178 ) ;
#7975=VERTEX_POINT ( 'NONE', #17801 ) ;
#7977=CARTESIAN_POINT ( 'NONE',  ( -10.00000000000000000, 16.59999999999999787, 2.499999999999998224 ) ) ;
#7982=ORIENTED_EDGE ( 'NONE', *, *, #5352, .T. ) ;
#7989=ORIENTED_EDGE ( 'NONE', *, *, #5422, .T. ) ;
#7991=DIRECTION ( 'NONE',  ( 1.000000000000000000, 0.000000000000000000, 0.000000000000000000 ) ) ;
#7994=ORIENTED_EDGE ( 'NONE', *, *, #18330, .T. ) ;
#7995=AXIS2_PLACEMENT_3D ( 'NONE', #15630, #1820, #11531 ) ;
#8004=DIRECTION ( 'NONE',  ( -0.000000000000000000, -1.000000000000000000, -0.000000000000000000 ) ) ;
#8007=CARTESIAN_POINT ( 'NONE',  ( 9.000000000000000000, 23.19999999999999574, -2.500000000000001332 ) ) ;
#8010=ORIENTED_EDGE ( 'NONE', *, *, #13846, .T. ) ;
#8011=EDGE_CURVE ( 'NONE', #3470, #9679, #13272, .T. ) ;
#8013=DIRECTION ( 'NONE',  ( 1.000000000000000000, 0.000000000000000000, 0.000000000000000000 ) ) ;
#8017=DIRECTION ( 'NONE',  ( 1.000000000000000000, 0.000000000000000000, -4.336808689942021680E-16 ) ) ;
#8018=PRODUCT_CONTEXT ( 'NONE', #3466, 'mechanical' ) ;
#8019=AXIS2_PLACEMENT_3D ( 'NONE', #10636, #7851, #16310 ) ;
#8030=EDGE_CURVE ( 'NONE', #12347, #10347, #6784, .T. ) ;
#8046=ORIENTED_EDGE ( 'NONE', *, *, #11787, .T. ) ;
#8054=PRODUCT_DEFINITION_FORMATION_WITH_SPECIFIED_SOURCE ( 'ANY', '', #1911, .NOT_KNOWN. ) ;
#8058=ORIENTED_EDGE ( 'NONE', *, *, #5520, .T. ) ;
#8063=EDGE_CURVE ( 'NONE', #13521, #3191, #4128, .T. ) ;
#8067=EDGE_CURVE ( 'NONE', #17010, #13521, #17171, .T. ) ;
#8070=ADVANCED_FACE ( 'NONE', ( #15367 ), #13299, .T. ) ;
#8072=STYLED_ITEM('',(#18396),#7822);
#8074=( NAMED_UNIT ( * ) SI_UNIT ( $, .STERADIAN. ) SOLID_ANGLE_UNIT ( ) );
#8083=DIRECTION ( 'NONE',  ( 0.000000000000000000, 0.000000000000000000, 1.000000000000000000 ) ) ;
#8092=FACE_OUTER_BOUND ( 'NONE', #12682, .T. ) ;
#8095=DIRECTION ( 'NONE',  ( 0.000000000000000000, 0.000000000000000000, -1.000000000000000000 ) ) ;
#8098=DIRECTION ( 'NONE',  ( -0.000000000000000000, -1.000000000000000000, -0.000000000000000000 ) ) ;
#8101=AXIS2_PLACEMENT_3D ( 'NONE', #9932, #10201, #15603 ) ;
#8104=DIRECTION ( 'NONE',  ( -3.469446951953613696E-16, -0.000000000000000000, -1.000000000000000000 ) ) ;
#8108=DIRECTION ( 'NONE',  ( -0.000000000000000000, -1.000000000000000000, -0.000000000000000000 ) ) ;
#8110=CYLINDRICAL_SURFACE ( 'NONE', #6898, 0.9999999999999991118 ) ;
#8113=UNCERTAINTY_MEASURE_WITH_UNIT (LENGTH_MEASURE( 1.000000000000000082E-05 ), #13700, 'distance_accuracy_value', 'NONE');
#8118=DIRECTION ( 'NONE',  ( -3.469446951953613696E-16, -0.000000000000000000, -1.000000000000000000 ) ) ;
#8134=ORIENTED_EDGE ( 'NONE', *, *, #11225, .T. ) ;
#8137=EDGE_CURVE ( 'NONE', #1200, #9609, #8908, .T. ) ;
#8141=DIRECTION ( 'NONE',  ( -0.000000000000000000, -1.000000000000000000, -0.000000000000000000 ) ) ;
#8149=CYLINDRICAL_SURFACE ( 'NONE', #4804, 0.9999999999999991118 ) ;
#8152=EDGE_LOOP ( 'NONE', ( #13396, #13900, #9530, #6124 ) ) ;
#8162=AXIS2_PLACEMENT_3D ( 'NONE', #15331, #15147, #9746 ) ;
#8167=ADVANCED_FACE ( 'NONE', ( #5519 ), #11164, .T. ) ;
#8171=ORIENTED_EDGE ( 'NONE', *, *, #13976, .F. ) ;
#8172=ORIENTED_EDGE ( 'NONE', *, *, #11787, .F. ) ;
#8173=CARTESIAN_POINT ( 'NONE',  ( 8.000000000000001776, 20.99999999999999289, -2.500000000000002220 ) ) ;
#8176=CARTESIAN_POINT ( 'NONE',  ( -10.00000000000000000, 40.79999999999999716, 2.499999999999998224 ) ) ;
#8183=TOROIDAL_SURFACE ( 'NONE', #8765, 9.000000000000001776, 0.9999999999999991118 ) ;
#8184=DIRECTION ( 'NONE',  ( 1.000000000000000000, 0.000000000000000000, -4.336808689942021680E-16 ) ) ;
#8187=ADVANCED_FACE ( 'NONE', ( #8301 ), #15718, .T. ) ;
#8199=MANIFOLD_SOLID_BREP ( 'LPattern6[7]', #226 ) ;
#8209=DIRECTION ( 'NONE',  ( -0.000000000000000000, -1.000000000000000000, -0.000000000000000000 ) ) ;
#8210=DIRECTION ( 'NONE',  ( -3.469446951953613696E-16, -0.000000000000000000, -1.000000000000000000 ) ) ;
#8211=DIRECTION ( 'NONE',  ( 0.000000000000000000, 0.000000000000000000, -1.000000000000000000 ) ) ;
#8223=CARTESIAN_POINT ( 'NONE',  ( -1.734723475976807094E-15, 18.79999999999999361, -11.50000000000000178 ) ) ;
#8226=ORIENTED_EDGE ( 'NONE', *, *, #802, .F. ) ;
#8234=AXIS2_PLACEMENT_3D ( 'NONE', #1325, #2537, #15242 ) ;
#8238=CARTESIAN_POINT ( 'NONE',  ( -9.000000000000003553, 20.99999999999999289, -2.500000000000001776 ) ) ;
#8241=ORIENTED_EDGE ( 'NONE', *, *, #4555, .T. ) ;
#8242=DIRECTION ( 'NONE',  ( -1.000000000000000000, 0.000000000000000000, 4.336808689942021680E-16 ) ) ;
#8244=EDGE_LOOP ( 'NONE', ( #9413, #6544, #6426, #12500 ) ) ;
#8253=CIRCLE ( 'NONE', #1704, 0.9999999999999991118 ) ;
#8260=DIRECTION ( 'NONE',  ( 0.000000000000000000, 0.000000000000000000, 1.000000000000000000 ) ) ;
#8265=EDGE_CURVE ( 'NONE', #18266, #16267, #2101, .T. ) ;
#8267=ADVANCED_FACE ( 'NONE', ( #8841 ), #2533, .T. ) ;
#8269=ORIENTED_EDGE ( 'NONE', *, *, #17528, .F. ) ;
#8270=CYLINDRICAL_SURFACE ( 'NONE', #4993, 0.9999999999999991118 ) ;
#8281=CARTESIAN_POINT ( 'NONE',  ( -1.734723475976807094E-15, 29.79999999999999716, -2.500000000000000000 ) ) ;
#8282=CARTESIAN_POINT ( 'NONE',  ( -10.00000000000000000, 34.19999999999999574, 2.499999999999998224 ) ) ;
#8301=FACE_OUTER_BOUND ( 'NONE', #18012, .T. ) ;
#8305=DIRECTION ( 'NONE',  ( -4.915049848600951133E-16, 0.000000000000000000, -1.000000000000000000 ) ) ;
#8306=DIRECTION ( 'NONE',  ( -0.000000000000000000, -1.000000000000000000, -0.000000000000000000 ) ) ;
#8322=ORIENTED_EDGE ( 'NONE', *, *, #14092, .T. ) ;
#8333=FACE_OUTER_BOUND ( 'NONE', #7668, .T. ) ;
#8343=CIRCLE ( 'NONE', #3615, 8.000000000000001776 ) ;
#8345=AXIS2_PLACEMENT_3D ( 'NONE', #6611, #16733, #15148 ) ;
#8348=DIRECTION ( 'NONE',  ( -3.469446951953613696E-16, -0.000000000000000000, -1.000000000000000000 ) ) ;
#8351=MANIFOLD_SOLID_BREP ( 'LPattern6[9]', #10285 ) ;
#8352=CARTESIAN_POINT ( 'NONE',  ( -9.000000000000001776, 18.79999999999999361, 2.499999999999995559 ) ) ;
#8353=FACE_OUTER_BOUND ( 'NONE', #9090, .T. ) ;
#8357=CARTESIAN_POINT ( 'NONE',  ( -1.734723475976807094E-15, 29.79999999999999716, -11.50000000000000178 ) ) ;
#8369=ADVANCED_FACE ( 'NONE', ( #3811 ), #1136, .T. ) ;
#8370=AXIS2_PLACEMENT_3D ( 'NONE', #6810, #5237, #8017 ) ;
#8372=DIRECTION ( 'NONE',  ( -4.915049848600951133E-16, 0.000000000000000000, -1.000000000000000000 ) ) ;
#8379=CIRCLE ( 'NONE', #1897, 0.9999999999999991118 ) ;
#8384=DIRECTION ( 'NONE',  ( 1.000000000000000000, 0.000000000000000000, -4.336808689942021680E-16 ) ) ;
#8397=PRODUCT_DEFINITION_CONTEXT ( 'detailed design', #630, 'design' ) ;
#8402=UNCERTAINTY_MEASURE_WITH_UNIT (LENGTH_MEASURE( 1.000000000000000082E-05 ), #15835, 'distance_accuracy_value', 'NONE');
#8407=EDGE_CURVE ( 'NONE', #5921, #15102, #6278, .T. ) ;
#8409=ORIENTED_EDGE ( 'NONE', *, *, #1512, .F. ) ;
#8414=ORIENTED_EDGE ( 'NONE', *, *, #2173, .T. ) ;
#8415=DIRECTION ( 'NONE',  ( -4.915049848600951133E-16, 0.000000000000000000, -1.000000000000000000 ) ) ;
#8428=ORIENTED_EDGE ( 'NONE', *, *, #131, .T. ) ;
#8439=CYLINDRICAL_SURFACE ( 'NONE', #7564, 0.9999999999999991118 ) ;
#8441=ORIENTED_EDGE ( 'NONE', *, *, #13744, .F. ) ;
#8449=AXIS2_PLACEMENT_3D ( 'NONE', #1843, #14735, #2034 ) ;
#8454=TOROIDAL_SURFACE ( 'NONE', #490, 9.000000000000001776, 0.9999999999999991118 ) ;
#8459=ADVANCED_FACE ( 'NONE', ( #5834 ), #15678, .T. ) ;
#8460=CIRCLE ( 'NONE', #12909, 0.9999999999999991118 ) ;
#8464=ORIENTED_EDGE ( 'NONE', *, *, #15238, .T. ) ;
#8467=DIRECTION ( 'NONE',  ( 0.000000000000000000, 0.000000000000000000, 1.000000000000000000 ) ) ;
#8468=AXIS2_PLACEMENT_3D ( 'NONE', #18050, #11147, #9580 ) ;
#8470=CARTESIAN_POINT ( 'NONE',  ( 9.000000000000005329, 18.79999999999999361, 2.499999999999997335 ) ) ;
#8488=ORIENTED_EDGE ( 'NONE', *, *, #12813, .F. ) ;
#8493=AXIS2_PLACEMENT_3D ( 'NONE', #168, #454, #3238 ) ;
#8494=DIRECTION ( 'NONE',  ( 0.000000000000000000, 0.000000000000000000, 1.000000000000000000 ) ) ;
#8495=AXIS2_PLACEMENT_3D ( 'NONE', #14239, #12469, #9871 ) ;
#8496=CARTESIAN_POINT ( 'NONE',  ( 9.000000000000001776, 27.59999999999999432, -2.500000000000002665 ) ) ;
#8500=ORIENTED_EDGE ( 'NONE', *, *, #18026, .T. ) ;
#8510=CIRCLE ( 'NONE', #12357, 0.9999999999999991118 ) ;
#8512=VERTEX_POINT ( 'NONE', #3703 ) ;
#8513=EDGE_CURVE ( 'NONE', #1278, #3449, #9350, .T. ) ;
#8514=CARTESIAN_POINT ( 'NONE',  ( 10.00000000000000355, 38.59999999999999432, 2.499999999999996891 ) ) ;
#8523=CARTESIAN_POINT ( 'NONE',  ( 0.000000000000000000, 34.19999999999999574, 2.500000000000000000 ) ) ;
#8525=AXIS2_PLACEMENT_3D ( 'NONE', #1900, #7530, #13183 ) ;
#8530=DIRECTION ( 'NONE',  ( -0.000000000000000000, -1.000000000000000000, -0.000000000000000000 ) ) ;
#8542=EDGE_CURVE ( 'NONE', #11668, #10052, #12559, .T. ) ;
#8543=DIRECTION ( 'NONE',  ( 0.000000000000000000, 0.000000000000000000, 1.000000000000000000 ) ) ;
#8547=( NAMED_UNIT ( * ) SI_UNIT ( $, .STERADIAN. ) SOLID_ANGLE_UNIT ( ) );
#8549=CIRCLE ( 'NONE', #13303, 10.00000000000000000 ) ;
#8553=CARTESIAN_POINT ( 'NONE',  ( 9.999999999999998224, 25.39999999999999503, -2.500000000000001776 ) ) ;
#8559=ADVANCED_FACE ( 'NONE', ( #10656 ), #17326, .T. ) ;
#8564=CARTESIAN_POINT ( 'NONE',  ( -1.734723475976807094E-15, 20.99999999999999289, -2.500000000000000000 ) ) ;
#8567=CARTESIAN_POINT ( 'NONE',  ( -1.734723475976807094E-15, 40.79999999999999716, -2.500000000000000000 ) ) ;
#8572=ORIENTED_EDGE ( 'NONE', *, *, #14532, .F. ) ;
#8574=CARTESIAN_POINT ( 'NONE',  ( -9.000000000000003553, 34.19999999999999574, -2.500000000000001776 ) ) ;
#8576=CIRCLE ( 'NONE', #7404, 0.9999999999999991118 ) ;
#8582=VERTEX_POINT ( 'NONE', #16328 ) ;
#8586=AXIS2_PLACEMENT_3D ( 'NONE', #18169, #11353, #12658 ) ;
#8594=VERTEX_POINT ( 'NONE', #14668 ) ;
#8595=CARTESIAN_POINT ( 'NONE',  ( -1.734723475976807094E-15, 25.39999999999999503, -2.500000000000000000 ) ) ;
#8603=DIRECTION ( 'NONE',  ( -3.373073425510457965E-16, 0.000000000000000000, -1.000000000000000000 ) ) ;
#8609=DIRECTION ( 'NONE',  ( 1.000000000000000000, 0.000000000000000000, 0.000000000000000000 ) ) ;
#8611=ORIENTED_EDGE ( 'NONE', *, *, #7508, .T. ) ;
#8615=( LENGTH_UNIT ( ) NAMED_UNIT ( * ) SI_UNIT ( .MILLI., .METRE. ) );
#8618=ORIENTED_EDGE ( 'NONE', *, *, #7106, .T. ) ;
#8630=CIRCLE ( 'NONE', #4217, 8.000000000000001776 ) ;
#8643=DIRECTION ( 'NONE',  ( 0.000000000000000000, 0.000000000000000000, -1.000000000000000000 ) ) ;
#8645=ORIENTED_EDGE ( 'NONE', *, *, #6159, .T. ) ;
#8653=DIRECTION ( 'NONE',  ( -0.000000000000000000, -1.000000000000000000, -0.000000000000000000 ) ) ;
#8659=( GEOMETRIC_REPRESENTATION_CONTEXT ( 3 ) GLOBAL_UNCERTAINTY_ASSIGNED_CONTEXT ( ( #2682 ) ) GLOBAL_UNIT_ASSIGNED_CONTEXT ( ( #8615, #1595, #10480 ) ) REPRESENTATION_CONTEXT ( 'NONE', 'WORKASPACE' ) );
#8663=DIRECTION ( 'NONE',  ( -1.000000000000000000, 0.000000000000000000, 4.336808689942021680E-16 ) ) ;
#8665=CARTESIAN_POINT ( 'NONE',  ( 0.000000000000000000, 29.79999999999999716, 2.500000000000000000 ) ) ;
#8671=CIRCLE ( 'NONE', #16999, 8.000000000000003553 ) ;
#8675=DIRECTION ( 'NONE',  ( -0.000000000000000000, -1.000000000000000000, -0.000000000000000000 ) ) ;
#8691=EDGE_LOOP ( 'NONE', ( #2180, #6289, #11639, #14849 ) ) ;
#8695=VERTEX_POINT ( 'NONE', #4059 ) ;
#8699=DIRECTION ( 'NONE',  ( -3.469446951953613696E-16, -0.000000000000000000, -1.000000000000000000 ) ) ;
#8703=ORIENTED_EDGE ( 'NONE', *, *, #5649, .F. ) ;
#8708=FACE_OUTER_BOUND ( 'NONE', #4245, .T. ) ;
#8722=ADVANCED_FACE ( 'NONE', ( #1207 ), #14650, .T. ) ;
#8723=CARTESIAN_POINT ( 'NONE',  ( -9.000000000000003553, 25.39999999999999503, -2.500000000000001776 ) ) ;
#8724=DIRECTION ( 'NONE',  ( 1.000000000000000000, 0.000000000000000000, 0.000000000000000000 ) ) ;
#8730=ORIENTED_EDGE ( 'NONE', *, *, #10501, .F. ) ;
#8735=DIRECTION ( 'NONE',  ( -0.000000000000000000, -1.000000000000000000, -0.000000000000000000 ) ) ;
#8743=DIRECTION ( 'NONE',  ( -3.469446951953613696E-16, -0.000000000000000000, -1.000000000000000000 ) ) ;
#8747=CARTESIAN_POINT ( 'NONE',  ( -9.000000000000003553, 36.39999999999999147, -2.500000000000001776 ) ) ;
#8759=CIRCLE ( 'NONE', #790, 0.9999999999999991118 ) ;
#8760=DIRECTION ( 'NONE',  ( 0.000000000000000000, 0.000000000000000000, -1.000000000000000000 ) ) ;
#8765=AXIS2_PLACEMENT_3D ( 'NONE', #3020, #8653, #17509 ) ;
#8776=CARTESIAN_POINT ( 'NONE',  ( -10.00000000000000000, 31.99999999999999289, 2.499999999999996003 ) ) ;
#8780=DIRECTION ( 'NONE',  ( -0.000000000000000000, -1.000000000000000000, -0.000000000000000000 ) ) ;
#8785=ORIENTED_EDGE ( 'NONE', *, *, #17114, .T. ) ;
#8791=CARTESIAN_POINT ( 'NONE',  ( 9.000000000000000000, 43.00000000000000000, -2.500000000000001332 ) ) ;
#8792=VECTOR ( 'NONE', #15746, 1000.000000000000000 ) ;
#8799=DIRECTION ( 'NONE',  ( -1.000000000000000000, 0.000000000000000000, 0.000000000000000000 ) ) ;
#8801=ORIENTED_EDGE ( 'NONE', *, *, #4949, .F. ) ;
#8822=CARTESIAN_POINT ( 'NONE',  ( -1.734723475976807094E-15, 36.39999999999999147, -2.500000000000000000 ) ) ;
#8828=CARTESIAN_POINT ( 'NONE',  ( 10.00000000000000000, 31.99999999999999289, -2.500000000000003109 ) ) ;
#8841=FACE_OUTER_BOUND ( 'NONE', #2450, .T. ) ;
#8844=CIRCLE ( 'NONE', #11502, 0.9999999999999991118 ) ;
#8846=CARTESIAN_POINT ( 'NONE',  ( -10.00000000000000178, 29.79999999999999716, -2.500000000000001776 ) ) ;
#8850=EDGE_LOOP ( 'NONE', ( #7884, #9066, #5654, #5536 ) ) ;
#8859=EDGE_LOOP ( 'NONE', ( #15250, #17834, #15000, #3152 ) ) ;
#8865=EDGE_CURVE ( 'NONE', #13697, #3107, #4310, .T. ) ;
#8868=DIRECTION ( 'NONE',  ( 0.000000000000000000, 0.000000000000000000, -1.000000000000000000 ) ) ;
#8875=CARTESIAN_POINT ( 'NONE',  ( -1.734723475976807094E-15, 34.19999999999999574, -2.500000000000000000 ) ) ;
#8876=CIRCLE ( 'NONE', #3272, 8.000000000000001776 ) ;
#8881=DIRECTION ( 'NONE',  ( 0.000000000000000000, 0.000000000000000000, -1.000000000000000000 ) ) ;
#8890=DIRECTION ( 'NONE',  ( -3.373073425510457965E-16, 0.000000000000000000, -1.000000000000000000 ) ) ;
#8901=CARTESIAN_POINT ( 'NONE',  ( 0.000000000000000000, 20.99999999999999289, 2.500000000000000000 ) ) ;
#8905=CARTESIAN_POINT ( 'NONE',  ( -1.734723475976807094E-15, 25.39999999999999503, -2.500000000000000000 ) ) ;
#8908=CIRCLE ( 'NONE', #7126, 0.9999999999999991118 ) ;
#8917=DIRECTION ( 'NONE',  ( -4.915049848600951133E-16, 0.000000000000000000, -1.000000000000000000 ) ) ;
#8920=CARTESIAN_POINT ( 'NONE',  ( -1.734723475976807094E-15, 18.79999999999999361, -2.500000000000000000 ) ) ;
#8922=ORIENTED_EDGE ( 'NONE', *, *, #15717, .F. ) ;
#8929=DIRECTION ( 'NONE',  ( 3.469446951953612217E-16, -0.000000000000000000, 1.000000000000000000 ) ) ;
#8930=EDGE_CURVE ( 'NONE', #3107, #13697, #16471, .T. ) ;
#8933=DIRECTION ( 'NONE',  ( -0.000000000000000000, -1.000000000000000000, -0.000000000000000000 ) ) ;
#8960=ORIENTED_EDGE ( 'NONE', *, *, #12288, .F. ) ;
#8961=DIRECTION ( 'NONE',  ( -1.000000000000000000, 0.000000000000000000, 4.336808689942021680E-16 ) ) ;
#8973=ORIENTED_EDGE ( 'NONE', *, *, #6778, .F. ) ;
#8978=ORIENTED_EDGE ( 'NONE', *, *, #5352, .F. ) ;
#8980=DIRECTION ( 'NONE',  ( 1.000000000000000000, 0.000000000000000000, 0.000000000000000000 ) ) ;
#8987=ORIENTED_EDGE ( 'NONE', *, *, #7959, .F. ) ;
#8992=DIRECTION ( 'NONE',  ( -0.000000000000000000, -1.000000000000000000, -0.000000000000000000 ) ) ;
#9002=CARTESIAN_POINT ( 'NONE',  ( -1.734723475976807094E-15, 36.39999999999999147, -2.500000000000000000 ) ) ;
#9003=CYLINDRICAL_SURFACE ( 'NONE', #7155, 0.9999999999999991118 ) ;
#9007=CARTESIAN_POINT ( 'NONE',  ( 9.000000000000005329, 29.79999999999999716, 2.499999999999997335 ) ) ;
#9017=VERTEX_POINT ( 'NONE', #15838 ) ;
#9024=CARTESIAN_POINT ( 'NONE',  ( 0.000000000000000000, 0.000000000000000000, 0.000000000000000000 ) ) ;
#9028=CARTESIAN_POINT ( 'NONE',  ( 0.000000000000000000, 27.59999999999999432, 2.500000000000000000 ) ) ;
#9035=CARTESIAN_POINT ( 'NONE',  ( 8.000000000000005329, 25.39999999999999503, 2.499999999999997780 ) ) ;
#9039=DIRECTION ( 'NONE',  ( 0.000000000000000000, 0.000000000000000000, -1.000000000000000000 ) ) ;
#9043=ORIENTED_EDGE ( 'NONE', *, *, #85, .T. ) ;
#9059=CARTESIAN_POINT ( 'NONE',  ( 10.00000000000000000, 38.59999999999999432, -2.500000000000003109 ) ) ;
#9066=ORIENTED_EDGE ( 'NONE', *, *, #15843, .T. ) ;
#9087=DIRECTION ( 'NONE',  ( -0.000000000000000000, -1.000000000000000000, -0.000000000000000000 ) ) ;
#9090=EDGE_LOOP ( 'NONE', ( #17618, #14196, #16794, #8058 ) ) ;
#9099=CIRCLE ( 'NONE', #1115, 8.000000000000003553 ) ;
#9106=AXIS2_PLACEMENT_3D ( 'NONE', #5331, #6194, #11844 ) ;
#9108=AXIS2_PLACEMENT_3D ( 'NONE', #14371, #1673, #4446 ) ;
#9109=ORIENTED_EDGE ( 'NONE', *, *, #16020, .T. ) ;
#9110=TOROIDAL_SURFACE ( 'NONE', #3493, 9.000000000000001776, 0.9999999999999991118 ) ;
#9111=ORIENTED_EDGE ( 'NONE', *, *, #16594, .T. ) ;
#9120=DIRECTION ( 'NONE',  ( -0.000000000000000000, -1.000000000000000000, -0.000000000000000000 ) ) ;
#9123=CIRCLE ( 'NONE', #16849, 0.9999999999999991118 ) ;
#9127=CARTESIAN_POINT ( 'NONE',  ( -10.00000000000000178, 36.39999999999999147, -2.500000000000001776 ) ) ;
#9128=CARTESIAN_POINT ( 'NONE',  ( -1.734723475976807094E-15, 29.79999999999999716, -2.500000000000000000 ) ) ;
#9130=ORIENTED_EDGE ( 'NONE', *, *, #31, .F. ) ;
#9134=CIRCLE ( 'NONE', #5874, 0.9999999999999991118 ) ;
#9142=EDGE_LOOP ( 'NONE', ( #17848, #11372, #15956, #14922 ) ) ;
#9145=EDGE_LOOP ( 'NONE', ( #7400, #7941, #17552, #7669 ) ) ;
#9149=CARTESIAN_POINT ( 'NONE',  ( 8.000000000000005329, 36.39999999999999147, 2.499999999999997780 ) ) ;
#9150=DIRECTION ( 'NONE',  ( -0.000000000000000000, -1.000000000000000000, -0.000000000000000000 ) ) ;
#9156=ORIENTED_EDGE ( 'NONE', *, *, #13115, .F. ) ;
#9160=ORIENTED_EDGE ( 'NONE', *, *, #8407, .T. ) ;
#9166=CIRCLE ( 'NONE', #1181, 0.9999999999999991118 ) ;
#9173=DIRECTION ( 'NONE',  ( -1.000000000000000000, 0.000000000000000000, 4.336808689942021680E-16 ) ) ;
#9180=VERTEX_POINT ( 'NONE', #11836 ) ;
#9182=CARTESIAN_POINT ( 'NONE',  ( -1.734723475976807094E-15, 20.99999999999999289, -2.500000000000000000 ) ) ;
#9183=DIRECTION ( 'NONE',  ( 1.000000000000000000, 0.000000000000000000, 0.000000000000000000 ) ) ;
#9185=ORIENTED_EDGE ( 'NONE', *, *, #1184, .F. ) ;
#9187=DIRECTION ( 'NONE',  ( -0.000000000000000000, -1.000000000000000000, -0.000000000000000000 ) ) ;
#9190=TOROIDAL_SURFACE ( 'NONE', #13633, 9.000000000000001776, 0.9999999999999991118 ) ;
#9198=CIRCLE ( 'NONE', #13042, 0.9999999999999991118 ) ;
#9200=ADVANCED_FACE ( 'NONE', ( #4886 ), #3724, .T. ) ;
#9203=ORIENTED_EDGE ( 'NONE', *, *, #17859, .T. ) ;
#9207=LINE ( 'NONE', #12165, #2035 ) ;
#9208=EDGE_CURVE ( 'NONE', #14942, #156, #14394, .T. ) ;
#9214=EDGE_CURVE ( 'NONE', #2806, #5635, #17383, .T. ) ;
#9216=CARTESIAN_POINT ( 'NONE',  ( -1.734723475976807094E-15, 16.59999999999999787, -2.500000000000000000 ) ) ;
#9222=CARTESIAN_POINT ( 'NONE',  ( -9.000000000000003553, 43.00000000000000000, -2.500000000000001776 ) ) ;
#9232=CARTESIAN_POINT ( 'NONE',  ( -8.000000000000001776, 29.79999999999999716, 2.499999999999995115 ) ) ;
#9233=EDGE_LOOP ( 'NONE', ( #4091, #17813, #5530, #7043 ) ) ;
#9234=CIRCLE ( 'NONE', #3030, 0.9999999999999991118 ) ;
#9238=ORIENTED_EDGE ( 'NONE', *, *, #14993, .F. ) ;
#9240=FACE_OUTER_BOUND ( 'NONE', #2400, .T. ) ;
#9245=ORIENTED_EDGE ( 'NONE', *, *, #10738, .T. ) ;
#9249=TOROIDAL_SURFACE ( 'NONE', #4521, 9.000000000000003553, 0.9999999999999991118 ) ;
#9251=EDGE_LOOP ( 'NONE', ( #8730, #10779, #2252, #3495 ) ) ;
#9264=CARTESIAN_POINT ( 'NONE',  ( 10.00000000000000000, 27.59999999999999432, -2.500000000000003109 ) ) ;
#9277=AXIS2_PLACEMENT_3D ( 'NONE', #9359, #13625, #15309 ) ;
#9279=CARTESIAN_POINT ( 'NONE',  ( 8.000000000000001776, 25.39999999999999503, -2.500000000000002220 ) ) ;
#9290=CARTESIAN_POINT ( 'NONE',  ( -1.734723475976807094E-15, 31.99999999999999289, -2.500000000000000000 ) ) ;
#9292=ORIENTED_EDGE ( 'NONE', *, *, #12355, .T. ) ;
#9301=CYLINDRICAL_SURFACE ( 'NONE', #14030, 0.9999999999999991118 ) ;
#9303=EDGE_CURVE ( 'NONE', #2685, #7975, #9645, .T. ) ;
#9314=CARTESIAN_POINT ( 'NONE',  ( 0.000000000000000000, 18.79999999999999361, 2.500000000000000000 ) ) ;
#9319=CARTESIAN_POINT ( 'NONE',  ( -8.000000000000003553, 23.19999999999999574, -2.500000000000001776 ) ) ;
#9320=FACE_OUTER_BOUND ( 'NONE', #3514, .T. ) ;
#9321=EDGE_CURVE ( 'NONE', #15889, #11926, #2565, .T. ) ;
#9323=EDGE_LOOP ( 'NONE', ( #14934, #7531, #14245, #16646 ) ) ;
#9326=EDGE_CURVE ( 'NONE', #12622, #10092, #12899, .T. ) ;
#9327=ORIENTED_EDGE ( 'NONE', *, *, #16722, .T. ) ;
#9328=( NAMED_UNIT ( * ) SI_UNIT ( $, .STERADIAN. ) SOLID_ANGLE_UNIT ( ) );
#9334=DIRECTION ( 'NONE',  ( 3.469446951953612217E-16, -0.000000000000000000, 1.000000000000000000 ) ) ;
#9345=AXIS2_PLACEMENT_3D ( 'NONE', #1561, #2782, #3045 ) ;
#9350=LINE ( 'NONE', #9264, #17315 ) ;
#9353=AXIS2_PLACEMENT_3D ( 'NONE', #5410, #2465, #6883 ) ;
#9359=CARTESIAN_POINT ( 'NONE',  ( -1.734723475976807094E-15, 43.00000000000000000, -2.500000000000000000 ) ) ;
#9362=EDGE_LOOP ( 'NONE', ( #4873, #325, #8241, #14764 ) ) ;
#9369=ORIENTED_EDGE ( 'NONE', *, *, #16096, .F. ) ;
#9375=DIRECTION ( 'NONE',  ( -1.000000000000000000, 0.000000000000000000, 4.336808689942021680E-16 ) ) ;
#9377=FACE_OUTER_BOUND ( 'NONE', #12136, .T. ) ;
#9378=VERTEX_POINT ( 'NONE', #4395 ) ;
#9381=CARTESIAN_POINT ( 'NONE',  ( -1.734723475976807094E-15, 43.00000000000000000, -12.50000000000000000 ) ) ;
#9383=EDGE_LOOP ( 'NONE', ( #15399, #8960, #10380, #15109 ) ) ;
#9391=AXIS2_PLACEMENT_3D ( 'NONE', #4252, #14076, #3978 ) ;
#9400=DIRECTION ( 'NONE',  ( -0.000000000000000000, -1.000000000000000000, -0.000000000000000000 ) ) ;
#9404=CLOSED_SHELL ( 'NONE', ( #8559, #3207, #13458, #13654, #12218, #9200, #10895, #4112, #15161, #1287 ) ) ;
#9405=CARTESIAN_POINT ( 'NONE',  ( 9.000000000000001776, 25.39999999999999503, -2.500000000000002665 ) ) ;
#9413=ORIENTED_EDGE ( 'NONE', *, *, #8011, .F. ) ;
#9415=FACE_OUTER_BOUND ( 'NONE', #14730, .T. ) ;
#9416=CARTESIAN_POINT ( 'NONE',  ( -1.734723475976807094E-15, 36.39999999999999147, -11.50000000000000178 ) ) ;
#9417=STYLED_ITEM('',(#18396),#14659);
#9419=CIRCLE ( 'NONE', #8525, 0.9999999999999991118 ) ;
#9428=ORIENTED_EDGE ( 'NONE', *, *, #15229, .T. ) ;
#9435=ADVANCED_FACE ( 'NONE', ( #16279 ), #1972, .T. ) ;
#9436=CIRCLE ( 'NONE', #5603, 8.000000000000003553 ) ;
#9442=EDGE_CURVE ( 'NONE', #3449, #4032, #3150, .T. ) ;
#9445=CIRCLE ( 'NONE', #1160, 8.000000000000001776 ) ;
#9450=CARTESIAN_POINT ( 'NONE',  ( -1.734723475976807094E-15, 38.59999999999999432, -2.500000000000000000 ) ) ;
#9455=ORIENTED_EDGE ( 'NONE', *, *, #9321, .T. ) ;
#9464=AXIS2_PLACEMENT_3D ( 'NONE', #9687, #3861, #5616 ) ;
#9465=DIRECTION ( 'NONE',  ( 1.000000000000000000, 0.000000000000000000, 0.000000000000000000 ) ) ;
#9469=DIRECTION ( 'NONE',  ( -1.000000000000000000, 0.000000000000000000, 4.336808689942021680E-16 ) ) ;
#9472=CARTESIAN_POINT ( 'NONE',  ( -1.734723475976807094E-15, 40.79999999999999716, -2.500000000000000000 ) ) ;
#9475=ORIENTED_EDGE ( 'NONE', *, *, #10152, .T. ) ;
#9487=CYLINDRICAL_SURFACE ( 'NONE', #3840, 0.9999999999999991118 ) ;
#9488=DIRECTION ( 'NONE',  ( -3.469446951953613696E-16, -0.000000000000000000, -1.000000000000000000 ) ) ;
#9494=ADVANCED_FACE ( 'NONE', ( #7818 ), #5508, .T. ) ;
#9497=DIRECTION ( 'NONE',  ( 3.469446951953612217E-16, -0.000000000000000000, 1.000000000000000000 ) ) ;
#9500=DIRECTION ( 'NONE',  ( 1.000000000000000000, 0.000000000000000000, -4.336808689942021680E-16 ) ) ;
#9521=UNCERTAINTY_MEASURE_WITH_UNIT (LENGTH_MEASURE( 1.000000000000000082E-05 ), #13827, 'distance_accuracy_value', 'NONE');
#9525=ORIENTED_EDGE ( 'NONE', *, *, #4447, .F. ) ;
#9530=ORIENTED_EDGE ( 'NONE', *, *, #2661, .T. ) ;
#9531=EDGE_CURVE ( 'NONE', #9655, #14197, #3160, .T. ) ;
#9549=AXIS2_PLACEMENT_3D ( 'NONE', #12300, #18261, #16409 ) ;
#9556=EDGE_CURVE ( 'NONE', #7574, #456, #13414, .T. ) ;
#9557=AXIS2_PLACEMENT_3D ( 'NONE', #13134, #16028, #8961 ) ;
#9566=ORIENTED_EDGE ( 'NONE', *, *, #4447, .T. ) ;
#9567=EDGE_LOOP ( 'NONE', ( #11004, #16157, #11698, #11865 ) ) ;
#9570=CARTESIAN_POINT ( 'NONE',  ( -1.734723475976807094E-15, 25.39999999999999503, -2.500000000000000000 ) ) ;
#9577=CARTESIAN_POINT ( 'NONE',  ( -1.734723475976807094E-15, 40.79999999999999716, -2.500000000000000000 ) ) ;
#9580=DIRECTION ( 'NONE',  ( -1.000000000000000000, 0.000000000000000000, 4.336808689942021680E-16 ) ) ;
#9583=FACE_OUTER_BOUND ( 'NONE', #5717, .T. ) ;
#9590=DIRECTION ( 'NONE',  ( -1.000000000000000000, 0.000000000000000000, 4.336808689942021680E-16 ) ) ;
#9596=ORIENTED_EDGE ( 'NONE', *, *, #18354, .T. ) ;
#9598=EDGE_CURVE ( 'NONE', #6179, #7574, #17398, .T. ) ;
#9600=EDGE_CURVE ( 'NONE', #17010, #15166, #16797, .T. ) ;
#9604=DIRECTION ( 'NONE',  ( 0.000000000000000000, 0.000000000000000000, -1.000000000000000000 ) ) ;
#9605=DIRECTION ( 'NONE',  ( 0.000000000000000000, 0.000000000000000000, -1.000000000000000000 ) ) ;
#9606=DIRECTION ( 'NONE',  ( 3.469446951953612217E-16, -0.000000000000000000, 1.000000000000000000 ) ) ;
#9607=DIRECTION ( 'NONE',  ( 0.000000000000000000, 0.000000000000000000, 1.000000000000000000 ) ) ;
#9609=VERTEX_POINT ( 'NONE', #12290 ) ;
#9627=VERTEX_POINT ( 'NONE', #2490 ) ;
#9629=ORIENTED_EDGE ( 'NONE', *, *, #18253, .F. ) ;
#9641=ORIENTED_EDGE ( 'NONE', *, *, #7106, .F. ) ;
#9645=CIRCLE ( 'NONE', #15576, 0.9999999999999991118 ) ;
#9649=VERTEX_POINT ( 'NONE', #12652 ) ;
#9651=DIRECTION ( 'NONE',  ( -0.000000000000000000, -1.000000000000000000, -0.000000000000000000 ) ) ;
#9652=ADVANCED_FACE ( 'NONE', ( #1452 ), #18278, .T. ) ;
#9653=CARTESIAN_POINT ( 'NONE',  ( 9.000000000000001776, 16.59999999999999787, -2.500000000000002665 ) ) ;
#9655=VERTEX_POINT ( 'NONE', #4307 ) ;
#9660=EDGE_CURVE ( 'NONE', #12347, #11426, #15020, .T. ) ;
#9665=ADVANCED_FACE ( 'NONE', ( #9782 ), #6907, .T. ) ;
#9675=CARTESIAN_POINT ( 'NONE',  ( -8.000000000000001776, 38.59999999999999432, 2.499999999999995115 ) ) ;
#9678=CARTESIAN_POINT ( 'NONE',  ( -8.000000000000001776, 29.79999999999999716, 2.499999999999998224 ) ) ;
#9679=VERTEX_POINT ( 'NONE', #5522 ) ;
#9682=AXIS2_PLACEMENT_3D ( 'NONE', #6667, #8415, #8242 ) ;
#9683=CIRCLE ( 'NONE', #16528, 8.000000000000001776 ) ;
#9687=CARTESIAN_POINT ( 'NONE',  ( 9.000000000000000000, 38.59999999999999432, -2.500000000000001332 ) ) ;
#9693=STYLED_ITEM('',(#18396),#13807);
#9701=EDGE_CURVE ( 'NONE', #9017, #14942, #186, .T. ) ;
#9702=ORIENTED_EDGE ( 'NONE', *, *, #13621, .T. ) ;
#9706=ORIENTED_EDGE ( 'NONE', *, *, #15424, .T. ) ;
#9707=( GEOMETRIC_REPRESENTATION_CONTEXT ( 3 ) GLOBAL_UNCERTAINTY_ASSIGNED_CONTEXT ( ( #18086 ) ) GLOBAL_UNIT_ASSIGNED_CONTEXT ( ( #109, #5670, #11053 ) ) REPRESENTATION_CONTEXT ( 'NONE', 'WORKASPACE' ) );
#9715=CARTESIAN_POINT ( 'NONE',  ( 0.000000000000000000, 23.19999999999999574, 2.500000000000000000 ) ) ;
#9739=AXIS2_PLACEMENT_3D ( 'NONE', #1964, #3345, #15957 ) ;
#9746=DIRECTION ( 'NONE',  ( 1.000000000000000000, 0.000000000000000000, -4.336808689942021680E-16 ) ) ;
#9751=AXIS2_PLACEMENT_3D ( 'NONE', #7552, #4871, #11818 ) ;
#9759=ADVANCED_FACE ( 'NONE', ( #1359 ), #10249, .T. ) ;
#9764=FACE_OUTER_BOUND ( 'NONE', #6241, .T. ) ;
#9771=DIRECTION ( 'NONE',  ( -3.469446951953613696E-16, -0.000000000000000000, -1.000000000000000000 ) ) ;
#9776=ORIENTED_EDGE ( 'NONE', *, *, #1453, .T. ) ;
#9780=DIRECTION ( 'NONE',  ( -1.000000000000000000, 0.000000000000000000, 4.336808689942021680E-16 ) ) ;
#9782=FACE_OUTER_BOUND ( 'NONE', #15243, .T. ) ;
#9785=ORIENTED_EDGE ( 'NONE', *, *, #1895, .F. ) ;
#9786=DIRECTION ( 'NONE',  ( 0.000000000000000000, 0.000000000000000000, -1.000000000000000000 ) ) ;
#9811=DIRECTION ( 'NONE',  ( -1.000000000000000000, 0.000000000000000000, 4.336808689942021680E-16 ) ) ;
#9819=EDGE_LOOP ( 'NONE', ( #14825, #2145, #17635, #3913 ) ) ;
#9827=EDGE_CURVE ( 'NONE', #1204, #8695, #8460, .T. ) ;
#9828=CARTESIAN_POINT ( 'NONE',  ( -1.734723475976807094E-15, 27.59999999999999432, -10.50000000000000178 ) ) ;
#9836=CARTESIAN_POINT ( 'NONE',  ( -1.734723475976807094E-15, 31.99999999999999289, -2.500000000000000000 ) ) ;
#9846=FACE_OUTER_BOUND ( 'NONE', #4142, .T. ) ;
#9847=CARTESIAN_POINT ( 'NONE',  ( 9.999999999999998224, 16.59999999999999787, -2.500000000000001776 ) ) ;
#9855=CARTESIAN_POINT ( 'NONE',  ( -10.00000000000000178, 18.79999999999999361, -2.500000000000001776 ) ) ;
#9860=AXIS2_PLACEMENT_3D ( 'NONE', #8223, #5446, #13887 ) ;
#9866=CARTESIAN_POINT ( 'NONE',  ( -1.734723475976807094E-15, 29.79999999999999716, -11.50000000000000178 ) ) ;
#9871=DIRECTION ( 'NONE',  ( 0.000000000000000000, 0.000000000000000000, -1.000000000000000000 ) ) ;
#9877=ORIENTED_EDGE ( 'NONE', *, *, #17903, .T. ) ;
#9879=ADVANCED_FACE ( 'NONE', ( #10230 ), #8183, .T. ) ;
#9895=ORIENTED_EDGE ( 'NONE', *, *, #7963, .T. ) ;
#9896=DIRECTION ( 'NONE',  ( -0.000000000000000000, -1.000000000000000000, -0.000000000000000000 ) ) ;
#9918=ORIENTED_EDGE ( 'NONE', *, *, #13173, .T. ) ;
#9932=CARTESIAN_POINT ( 'NONE',  ( -9.000000000000001776, 23.19999999999999574, 2.499999999999995559 ) ) ;
#9944=AXIS2_PLACEMENT_3D ( 'NONE', #9416, #10994, #15094 ) ;
#9946=CARTESIAN_POINT ( 'NONE',  ( 8.000000000000001776, 31.99999999999999289, -2.500000000000002220 ) ) ;
#9947=ADVANCED_FACE ( 'NONE', ( #614 ), #7283, .T. ) ;
#9952=( NAMED_UNIT ( * ) SI_UNIT ( $, .STERADIAN. ) SOLID_ANGLE_UNIT ( ) );
#9955=DIRECTION ( 'NONE',  ( -4.915049848600951133E-16, 0.000000000000000000, -1.000000000000000000 ) ) ;
#9960=DIRECTION ( 'NONE',  ( -3.373073425510457965E-16, 0.000000000000000000, -1.000000000000000000 ) ) ;
#9963=VERTEX_POINT ( 'NONE', #11624 ) ;
#9966=AXIS2_PLACEMENT_3D ( 'NONE', #14453, #10538, #3418 ) ;
#9968=ORIENTED_EDGE ( 'NONE', *, *, #1923, .T. ) ;
#9975=VECTOR ( 'NONE', #4611, 1000.000000000000000 ) ;
#9976=CARTESIAN_POINT ( 'NONE',  ( 0.000000000000000000, 31.99999999999999289, 2.500000000000000000 ) ) ;
#9977=EDGE_CURVE ( 'NONE', #17729, #16267, #3746, .T. ) ;
#9978=CIRCLE ( 'NONE', #14758, 0.9999999999999991118 ) ;
#9983=CARTESIAN_POINT ( 'NONE',  ( -9.000000000000001776, 34.19999999999999574, 2.499999999999995559 ) ) ;
#9992=ORIENTED_EDGE ( 'NONE', *, *, #15884, .F. ) ;
#9993=AXIS2_PLACEMENT_3D ( 'NONE', #10310, #11514, #11610 ) ;
#9995=AXIS2_PLACEMENT_3D ( 'NONE', #10405, #13281, #213 ) ;
#10004=CIRCLE ( 'NONE', #12368, 10.00000000000000000 ) ;
#10014=EDGE_LOOP ( 'NONE', ( #11962, #14852, #6595, #10168 ) ) ;
#10028=DIRECTION ( 'NONE',  ( 0.000000000000000000, 0.000000000000000000, 1.000000000000000000 ) ) ;
#10029=ORIENTED_EDGE ( 'NONE', *, *, #16027, .F. ) ;
#10030=AXIS2_PLACEMENT_3D ( 'NONE', #1945, #8675, #1652 ) ;
#10034=CARTESIAN_POINT ( 'NONE',  ( -1.734723475976807094E-15, 16.59999999999999787, -2.500000000000000000 ) ) ;
#10040=CIRCLE ( 'NONE', #2391, 0.9999999999999991118 ) ;
#10041=DIRECTION ( 'NONE',  ( -1.000000000000000000, 0.000000000000000000, 0.000000000000000000 ) ) ;
#10052=VERTEX_POINT ( 'NONE', #17782 ) ;
#10057=MECHANICAL_DESIGN_GEOMETRIC_PRESENTATION_REPRESENTATION('',(#18102),#17202);
#10064=ADVANCED_FACE ( 'NONE', ( #10789 ), #15896, .T. ) ;
#10073=ORIENTED_EDGE ( 'NONE', *, *, #2210, .T. ) ;
#10074=ORIENTED_EDGE ( 'NONE', *, *, #12523, .T. ) ;
#10091=EDGE_LOOP ( 'NONE', ( #12437, #5540, #5402, #6518 ) ) ;
#10092=VERTEX_POINT ( 'NONE', #11906 ) ;
#10106=AXIS2_PLACEMENT_3D ( 'NONE', #4938, #2182, #10594 ) ;
#10109=FACE_OUTER_BOUND ( 'NONE', #6680, .T. ) ;
#10113=DIRECTION ( 'NONE',  ( -0.000000000000000000, -1.000000000000000000, -0.000000000000000000 ) ) ;
#10114=VECTOR ( 'NONE', #16293, 1000.000000000000000 ) ;
#10116=CIRCLE ( 'NONE', #5090, 0.9999999999999991118 ) ;
#10121=ORIENTED_EDGE ( 'NONE', *, *, #4978, .F. ) ;
#10127=CARTESIAN_POINT ( 'NONE',  ( -1.734723475976807094E-15, 27.59999999999999432, -2.500000000000000000 ) ) ;
#10129=VECTOR ( 'NONE', #942, 1000.000000000000000 ) ;
#10132=CIRCLE ( 'NONE', #2754, 0.9999999999999991118 ) ;
#10138=DIRECTION ( 'NONE',  ( 1.000000000000000000, 0.000000000000000000, 0.000000000000000000 ) ) ;
#10146=ORIENTED_EDGE ( 'NONE', *, *, #4781, .F. ) ;
#10152=EDGE_CURVE ( 'NONE', #1108, #10845, #4338, .T. ) ;
#10167=CYLINDRICAL_SURFACE ( 'NONE', #18320, 0.9999999999999991118 ) ;
#10168=ORIENTED_EDGE ( 'NONE', *, *, #8265, .F. ) ;
#10176=EDGE_CURVE ( 'NONE', #4921, #4547, #11150, .T. ) ;
#10196=DIRECTION ( 'NONE',  ( 0.000000000000000000, 0.000000000000000000, 1.000000000000000000 ) ) ;
#10201=DIRECTION ( 'NONE',  ( -3.469446951953613696E-16, -0.000000000000000000, -1.000000000000000000 ) ) ;
#10203=DIRECTION ( 'NONE',  ( 3.469446951953612217E-16, -0.000000000000000000, 1.000000000000000000 ) ) ;
#10206=LINE ( 'NONE', #4653, #12443 ) ;
#10210=EDGE_LOOP ( 'NONE', ( #12601, #15209, #5934, #17265 ) ) ;
#10220=EDGE_CURVE ( 'NONE', #5429, #11926, #12920, .T. ) ;
#10221=DIRECTION ( 'NONE',  ( 0.000000000000000000, 0.000000000000000000, 1.000000000000000000 ) ) ;
#10222=CARTESIAN_POINT ( 'NONE',  ( -1.734723475976807094E-15, 23.19999999999999574, -2.500000000000000000 ) ) ;
#10223=ORIENTED_EDGE ( 'NONE', *, *, #375, .F. ) ;
#10226=AXIS2_PLACEMENT_3D ( 'NONE', #7844, #18069, #15091 ) ;
#10230=FACE_OUTER_BOUND ( 'NONE', #6477, .T. ) ;
#10241=FACE_OUTER_BOUND ( 'NONE', #16884, .T. ) ;
#10246=ORIENTED_EDGE ( 'NONE', *, *, #13173, .F. ) ;
#10249=TOROIDAL_SURFACE ( 'NONE', #2575, 9.000000000000001776, 0.9999999999999991118 ) ;
#10252=CARTESIAN_POINT ( 'NONE',  ( 0.000000000000000000, 38.59999999999999432, 2.500000000000000000 ) ) ;
#10254=DIRECTION ( 'NONE',  ( -1.000000000000000000, 0.000000000000000000, 0.000000000000000000 ) ) ;
#10258=ORIENTED_EDGE ( 'NONE', *, *, #1512, .T. ) ;
#10262=AXIS2_PLACEMENT_3D ( 'NONE', #10771, #2265, #6509 ) ;
#10263=ORIENTED_EDGE ( 'NONE', *, *, #9214, .T. ) ;
#10265=ADVANCED_FACE ( 'NONE', ( #16839 ), #14419, .T. ) ;
#10266=DIRECTION ( 'NONE',  ( 3.469446951953612217E-16, -0.000000000000000000, 1.000000000000000000 ) ) ;
#10273=ORIENTED_EDGE ( 'NONE', *, *, #14901, .F. ) ;
#10282=ADVANCED_FACE ( 'NONE', ( #16746 ), #15346, .T. ) ;
#10285=CLOSED_SHELL ( 'NONE', ( #13280, #7334, #3834, #15791, #6268, #7840, #12471, #5681, #6039, #6719 ) ) ;
#10286=CARTESIAN_POINT ( 'NONE',  ( 0.000000000000000000, 29.79999999999999716, 2.500000000000000000 ) ) ;
#10287=FACE_OUTER_BOUND ( 'NONE', #7088, .T. ) ;
#10290=ORIENTED_EDGE ( 'NONE', *, *, #11021, .F. ) ;
#10291=AXIS2_PLACEMENT_3D ( 'NONE', #15429, #2727, #14020 ) ;
#10301=DIRECTION ( 'NONE',  ( 0.000000000000000000, 0.000000000000000000, 1.000000000000000000 ) ) ;
#10305=CARTESIAN_POINT ( 'NONE',  ( -1.734723475976807094E-15, 31.99999999999999289, -2.500000000000000000 ) ) ;
#10310=CARTESIAN_POINT ( 'NONE',  ( 9.000000000000001776, 38.59999999999999432, -2.500000000000002665 ) ) ;
#10316=DIRECTION ( 'NONE',  ( 3.469446951953612217E-16, -0.000000000000000000, 1.000000000000000000 ) ) ;
#10317=CIRCLE ( 'NONE', #9682, 0.9999999999999991118 ) ;
#10318=CARTESIAN_POINT ( 'NONE',  ( -9.000000000000001776, 18.79999999999999361, 2.499999999999998224 ) ) ;
#10319=EDGE_CURVE ( 'NONE', #15990, #10466, #3177, .T. ) ;
#10320=EDGE_LOOP ( 'NONE', ( #4657, #7218, #7920, #14990 ) ) ;
#10325=DIRECTION ( 'NONE',  ( 1.000000000000000000, 0.000000000000000000, 0.000000000000000000 ) ) ;
#10327=AXIS2_PLACEMENT_3D ( 'NONE', #9976, #12680, #11103 ) ;
#10332=CYLINDRICAL_SURFACE ( 'NONE', #9751, 0.9999999999999991118 ) ;
#10347=VERTEX_POINT ( 'NONE', #29 ) ;
#10355=ORIENTED_EDGE ( 'NONE', *, *, #4911, .F. ) ;
#10357=( NAMED_UNIT ( * ) SI_UNIT ( $, .STERADIAN. ) SOLID_ANGLE_UNIT ( ) );
#10358=CIRCLE ( 'NONE', #2680, 0.9999999999999991118 ) ;
#10372=ORIENTED_EDGE ( 'NONE', *, *, #4495, .F. ) ;
#10380=ORIENTED_EDGE ( 'NONE', *, *, #11179, .T. ) ;
#10386=ORIENTED_EDGE ( 'NONE', *, *, #17640, .F. ) ;
#10400=LINE ( 'NONE', #11600, #15451 ) ;
#10401=CIRCLE ( 'NONE', #1825, 10.00000000000000000 ) ;
#10405=CARTESIAN_POINT ( 'NONE',  ( -9.000000000000003553, 18.79999999999999361, -2.500000000000001776 ) ) ;
#10407=EDGE_LOOP ( 'NONE', ( #17548, #1380, #14953, #9785 ) ) ;
#10409=FACE_OUTER_BOUND ( 'NONE', #13034, .T. ) ;
#10415=CARTESIAN_POINT ( 'NONE',  ( 9.000000000000001776, 23.19999999999999574, -2.500000000000002665 ) ) ;
#10419=CIRCLE ( 'NONE', #17568, 0.9999999999999991118 ) ;
#10428=DIRECTION ( 'NONE',  ( -0.000000000000000000, -1.000000000000000000, -0.000000000000000000 ) ) ;
#10430=LINE ( 'NONE', #9675, #12671 ) ;
#10432=ADVANCED_FACE ( 'NONE', ( #3372 ), #7003, .T. ) ;
#10438=DIRECTION ( 'NONE',  ( 0.000000000000000000, 0.000000000000000000, -1.000000000000000000 ) ) ;
#10445=CARTESIAN_POINT ( 'NONE',  ( -8.000000000000003553, 40.79999999999999716, -2.500000000000001776 ) ) ;
#10449=LINE ( 'NONE', #9059, #1179 ) ;
#10457=EDGE_CURVE ( 'NONE', #16267, #15166, #809, .T. ) ;
#10461=EDGE_CURVE ( 'NONE', #8594, #2439, #4646, .T. ) ;
#10466=VERTEX_POINT ( 'NONE', #7430 ) ;
#10480=( NAMED_UNIT ( * ) SI_UNIT ( $, .STERADIAN. ) SOLID_ANGLE_UNIT ( ) );
#10481=CARTESIAN_POINT ( 'NONE',  ( -9.000000000000001776, 16.59999999999999787, 2.499999999999995559 ) ) ;
#10488=EDGE_CURVE ( 'NONE', #1681, #8512, #15602, .T. ) ;
#10493=DIRECTION ( 'NONE',  ( -0.000000000000000000, -1.000000000000000000, -0.000000000000000000 ) ) ;
#10494=DIRECTION ( 'NONE',  ( -3.469446951953613696E-16, -0.000000000000000000, -1.000000000000000000 ) ) ;
#10496=DIRECTION ( 'NONE',  ( -0.000000000000000000, -1.000000000000000000, -0.000000000000000000 ) ) ;
#10498=ORIENTED_EDGE ( 'NONE', *, *, #238, .F. ) ;
#10501=EDGE_CURVE ( 'NONE', #15166, #3191, #15320, .T. ) ;
#10504=ORIENTED_EDGE ( 'NONE', *, *, #1293, .F. ) ;
#10513=DIRECTION ( 'NONE',  ( -0.000000000000000000, -1.000000000000000000, -0.000000000000000000 ) ) ;
#10516=DIRECTION ( 'NONE',  ( -0.000000000000000000, -1.000000000000000000, -0.000000000000000000 ) ) ;
#10521=CARTESIAN_POINT ( 'NONE',  ( -1.734723475976807094E-15, 31.99999999999999289, -2.500000000000000000 ) ) ;
#10524=ORIENTED_EDGE ( 'NONE', *, *, #4650, .F. ) ;
#10533=AXIS2_PLACEMENT_3D ( 'NONE', #11341, #9651, #6783 ) ;
#10538=DIRECTION ( 'NONE',  ( -0.000000000000000000, -1.000000000000000000, -0.000000000000000000 ) ) ;
#10544=ORIENTED_EDGE ( 'NONE', *, *, #2661, .F. ) ;
#10546=DIRECTION ( 'NONE',  ( 0.000000000000000000, 0.000000000000000000, 1.000000000000000000 ) ) ;
#10547=FILL_AREA_STYLE_COLOUR ( '', #2444 ) ;
#10552=ORIENTED_EDGE ( 'NONE', *, *, #8542, .F. ) ;
#10556=EDGE_CURVE ( 'NONE', #5725, #5839, #5534, .T. ) ;
#10569=CARTESIAN_POINT ( 'NONE',  ( -10.00000000000000178, 23.19999999999999574, -2.500000000000001776 ) ) ;
#10574=DIRECTION ( 'NONE',  ( -0.000000000000000000, -1.000000000000000000, -0.000000000000000000 ) ) ;
#10577=EDGE_CURVE ( 'NONE', #3191, #9017, #14691, .T. ) ;
#10585=CLOSED_SHELL ( 'NONE', ( #12149, #2330, #12874, #2820, #382, #12914, #17574, #11917, #4164, #8187 ) ) ;
#10588=MECHANICAL_DESIGN_GEOMETRIC_PRESENTATION_REPRESENTATION('',(#2021),#4363);
#10594=DIRECTION ( 'NONE',  ( 1.000000000000000000, 0.000000000000000000, -4.336808689942021680E-16 ) ) ;
#10595=DIRECTION ( 'NONE',  ( -0.000000000000000000, -1.000000000000000000, -0.000000000000000000 ) ) ;
#10605=AXIS2_PLACEMENT_3D ( 'NONE', #16749, #1256, #6890 ) ;
#10614=CIRCLE ( 'NONE', #15370, 8.000000000000001776 ) ;
#10616=AXIS2_PLACEMENT_3D ( 'NONE', #4356, #14573, #11674 ) ;
#10619=DIRECTION ( 'NONE',  ( 1.000000000000000000, 0.000000000000000000, -4.336808689942021680E-16 ) ) ;
#10620=SHAPE_DEFINITION_REPRESENTATION ( #17461, #7684 ) ;
#10622=ORIENTED_EDGE ( 'NONE', *, *, #2209, .F. ) ;
#10624=ADVANCED_FACE ( 'NONE', ( #17579 ), #685, .T. ) ;
#10629=DIRECTION ( 'NONE',  ( -0.000000000000000000, -1.000000000000000000, -0.000000000000000000 ) ) ;
#10633=EDGE_CURVE ( 'NONE', #4165, #14197, #7295, .T. ) ;
#10636=CARTESIAN_POINT ( 'NONE',  ( 9.000000000000000000, 27.59999999999999432, -2.500000000000001332 ) ) ;
#10637=AXIS2_PLACEMENT_3D ( 'NONE', #232, #7261, #5788 ) ;
#10641=DIRECTION ( 'NONE',  ( -0.000000000000000000, -1.000000000000000000, -0.000000000000000000 ) ) ;
#10654=CARTESIAN_POINT ( 'NONE',  ( 9.000000000000000000, 40.79999999999999716, -2.500000000000001332 ) ) ;
#10656=FACE_OUTER_BOUND ( 'NONE', #6555, .T. ) ;
#10661=ORIENTED_EDGE ( 'NONE', *, *, #18330, .F. ) ;
#10664=FACE_OUTER_BOUND ( 'NONE', #8244, .T. ) ;
#10666=ORIENTED_EDGE ( 'NONE', *, *, #6834, .F. ) ;
#10674=EDGE_LOOP ( 'NONE', ( #2415, #7982, #2119, #14945 ) ) ;
#10678=VECTOR ( 'NONE', #9334, 1000.000000000000000 ) ;
#10682=ORIENTED_EDGE ( 'NONE', *, *, #13846, .F. ) ;
#10683=CYLINDRICAL_SURFACE ( 'NONE', #18047, 0.9999999999999991118 ) ;
#10684=EDGE_CURVE ( 'NONE', #6854, #1143, #6429, .T. ) ;
#10686=DIRECTION ( 'NONE',  ( 0.000000000000000000, 0.000000000000000000, -1.000000000000000000 ) ) ;
#10699=FACE_OUTER_BOUND ( 'NONE', #13747, .T. ) ;
#10700=CARTESIAN_POINT ( 'NONE',  ( -10.00000000000000000, 38.59999999999999432, 2.499999999999996003 ) ) ;
#10704=CARTESIAN_POINT ( 'NONE',  ( -10.00000000000000000, 34.19999999999999574, 2.499999999999996003 ) ) ;
#10710=DIRECTION ( 'NONE',  ( -0.000000000000000000, -1.000000000000000000, -0.000000000000000000 ) ) ;
#10712=VECTOR ( 'NONE', #15805, 1000.000000000000000 ) ;
#10714=ADVANCED_FACE ( 'NONE', ( #11459 ), #11043, .T. ) ;
#10718=ORIENTED_EDGE ( 'NONE', *, *, #11537, .F. ) ;
#10726=DIRECTION ( 'NONE',  ( -1.000000000000000000, 0.000000000000000000, 4.336808689942021680E-16 ) ) ;
#10733=DIRECTION ( 'NONE',  ( -3.373073425510457965E-16, 0.000000000000000000, -1.000000000000000000 ) ) ;
#10735=SURFACE_SIDE_STYLE ('',( #13428 ) ) ;
#10738=EDGE_CURVE ( 'NONE', #5725, #2406, #13737, .T. ) ;
#10745=DIRECTION ( 'NONE',  ( -0.000000000000000000, -1.000000000000000000, -0.000000000000000000 ) ) ;
#10752=ORIENTED_EDGE ( 'NONE', *, *, #14417, .F. ) ;
#10760=DIRECTION ( 'NONE',  ( -1.000000000000000000, 0.000000000000000000, 0.000000000000000000 ) ) ;
#10769=CIRCLE ( 'NONE', #2790, 0.9999999999999991118 ) ;
#10771=CARTESIAN_POINT ( 'NONE',  ( -1.734723475976807094E-15, 43.00000000000000000, -2.500000000000000000 ) ) ;
#10779=ORIENTED_EDGE ( 'NONE', *, *, #9600, .F. ) ;
#10786=CIRCLE ( 'NONE', #11366, 0.9999999999999991118 ) ;
#10789=FACE_OUTER_BOUND ( 'NONE', #11998, .T. ) ;
#10799=DIRECTION ( 'NONE',  ( -1.000000000000000000, 0.000000000000000000, 4.336808689942021680E-16 ) ) ;
#10802=DIRECTION ( 'NONE',  ( -1.000000000000000000, 0.000000000000000000, 0.000000000000000000 ) ) ;
#10812=CYLINDRICAL_SURFACE ( 'NONE', #17777, 0.9999999999999991118 ) ;
#10817=ORIENTED_EDGE ( 'NONE', *, *, #477, .T. ) ;
#10818=DIRECTION ( 'NONE',  ( -0.000000000000000000, -1.000000000000000000, -0.000000000000000000 ) ) ;
#10832=ORIENTED_EDGE ( 'NONE', *, *, #8067, .F. ) ;
#10839=EDGE_LOOP ( 'NONE', ( #15430, #3697, #17183, #10029 ) ) ;
#10845=VERTEX_POINT ( 'NONE', #1565 ) ;
#10855=EDGE_CURVE ( 'NONE', #5429, #10347, #165, .T. ) ;
#10862=CARTESIAN_POINT ( 'NONE',  ( -1.734723475976807094E-15, 23.19999999999999574, -2.500000000000000000 ) ) ;
#10865=DIRECTION ( 'NONE',  ( 3.469446951953612217E-16, -0.000000000000000000, 1.000000000000000000 ) ) ;
#10878=AXIS2_PLACEMENT_3D ( 'NONE', #9715, #9896, #11284 ) ;
#10884=DIRECTION ( 'NONE',  ( 1.000000000000000000, 0.000000000000000000, -4.336808689942021680E-16 ) ) ;
#10888=DIRECTION ( 'NONE',  ( -3.469446951953613696E-16, -0.000000000000000000, -1.000000000000000000 ) ) ;
#10892=FACE_OUTER_BOUND ( 'NONE', #3187, .T. ) ;
#10895=ADVANCED_FACE ( 'NONE', ( #4522 ), #3478, .T. ) ;
#10905=DIRECTION ( 'NONE',  ( 0.000000000000000000, 0.000000000000000000, -1.000000000000000000 ) ) ;
#10908=CIRCLE ( 'NONE', #9995, 0.9999999999999991118 ) ;
#10927=CARTESIAN_POINT ( 'NONE',  ( -1.734723475976807094E-15, 23.19999999999999574, -2.500000000000000000 ) ) ;
#10933=ADVANCED_FACE ( 'NONE', ( #17628 ), #18006, .T. ) ;
#10935=ORIENTED_EDGE ( 'NONE', *, *, #16832, .T. ) ;
#10946=ORIENTED_EDGE ( 'NONE', *, *, #238, .T. ) ;
#10957=ORIENTED_EDGE ( 'NONE', *, *, #7103, .F. ) ;
#10963=ORIENTED_EDGE ( 'NONE', *, *, #12653, .T. ) ;
#10975=TOROIDAL_SURFACE ( 'NONE', #4174, 9.000000000000001776, 0.9999999999999991118 ) ;
#10978=DIRECTION ( 'NONE',  ( -0.000000000000000000, -1.000000000000000000, -0.000000000000000000 ) ) ;
#10982=CARTESIAN_POINT ( 'NONE',  ( -1.734723475976807094E-15, 38.59999999999999432, -10.50000000000000178 ) ) ;
#10994=DIRECTION ( 'NONE',  ( -1.000000000000000000, 0.000000000000000000, 0.000000000000000000 ) ) ;
#10995=STYLED_ITEM ( 'NONE', ( #17899 ), #18244 ) ;
#11004=ORIENTED_EDGE ( 'NONE', *, *, #1119, .F. ) ;
#11010=( GEOMETRIC_REPRESENTATION_CONTEXT ( 3 ) GLOBAL_UNCERTAINTY_ASSIGNED_CONTEXT ( ( #16852 ) ) GLOBAL_UNIT_ASSIGNED_CONTEXT ( ( #3873, #828, #6292 ) ) REPRESENTATION_CONTEXT ( 'NONE', 'WORKASPACE' ) );
#11013=ORIENTED_EDGE ( 'NONE', *, *, #6552, .F. ) ;
#11014=DIRECTION ( 'NONE',  ( 0.000000000000000000, 0.000000000000000000, -1.000000000000000000 ) ) ;
#11017=DIRECTION ( 'NONE',  ( 1.000000000000000000, 0.000000000000000000, 0.000000000000000000 ) ) ;
#11021=EDGE_CURVE ( 'NONE', #1567, #5909, #7308, .T. ) ;
#11022=CARTESIAN_POINT ( 'NONE',  ( -9.000000000000001776, 29.79999999999999716, 2.499999999999995559 ) ) ;
#11023=EDGE_LOOP ( 'NONE', ( #12534, #9877, #18304, #17003 ) ) ;
#11033=AXIS2_PLACEMENT_3D ( 'NONE', #13579, #15270, #16474 ) ;
#11037=EDGE_LOOP ( 'NONE', ( #4099, #10552, #8618, #466 ) ) ;
#11043=CYLINDRICAL_SURFACE ( 'NONE', #7910, 0.9999999999999991118 ) ;
#11046=AXIS2_PLACEMENT_3D ( 'NONE', #9182, #17467, #2158 ) ;
#11049=EDGE_LOOP ( 'NONE', ( #16313, #11112, #16810, #9776 ) ) ;
#11050=DIRECTION ( 'NONE',  ( 1.000000000000000000, 0.000000000000000000, -4.336808689942021680E-16 ) ) ;
#11053=( NAMED_UNIT ( * ) SI_UNIT ( $, .STERADIAN. ) SOLID_ANGLE_UNIT ( ) );
#11060=CARTESIAN_POINT ( 'NONE',  ( -9.000000000000001776, 40.79999999999999716, 2.499999999999995559 ) ) ;
#11064=EDGE_CURVE ( 'NONE', #5475, #1278, #13235, .T. ) ;
#11083=CARTESIAN_POINT ( 'NONE',  ( -10.00000000000000000, 43.00000000000000000, 2.499999999999998224 ) ) ;
#11085=VERTEX_POINT ( 'NONE', #1004 ) ;
#11099=ORIENTED_EDGE ( 'NONE', *, *, #16832, .F. ) ;
#11103=DIRECTION ( 'NONE',  ( 0.000000000000000000, 0.000000000000000000, -1.000000000000000000 ) ) ;
#11110=DIRECTION ( 'NONE',  ( -1.000000000000000000, 0.000000000000000000, 4.336808689942021680E-16 ) ) ;
#11112=ORIENTED_EDGE ( 'NONE', *, *, #12728, .F. ) ;
#11117=EDGE_CURVE ( 'NONE', #13534, #3470, #1425, .T. ) ;
#11126=CARTESIAN_POINT ( 'NONE',  ( -9.000000000000003553, 40.79999999999999716, -2.500000000000001776 ) ) ;
#11127=EDGE_CURVE ( 'NONE', #15647, #5839, #9683, .T. ) ;
#11129=AXIS2_PLACEMENT_3D ( 'NONE', #9216, #9120, #3389 ) ;
#11133=ORIENTED_EDGE ( 'NONE', *, *, #4387, .T. ) ;
#11134=CARTESIAN_POINT ( 'NONE',  ( 9.000000000000001776, 31.99999999999999289, -2.500000000000002665 ) ) ;
#11136=CARTESIAN_POINT ( 'NONE',  ( 9.000000000000001776, 29.79999999999999716, -2.500000000000002665 ) ) ;
#11145=DIRECTION ( 'NONE',  ( -3.469446951953613696E-16, -0.000000000000000000, -1.000000000000000000 ) ) ;
#11147=DIRECTION ( 'NONE',  ( -3.373073425510457965E-16, 0.000000000000000000, -1.000000000000000000 ) ) ;
#11150=CIRCLE ( 'NONE', #16502, 10.00000000000000178 ) ;
#11155=CARTESIAN_POINT ( 'NONE',  ( -9.000000000000001776, 27.59999999999999432, 2.499999999999995559 ) ) ;
#11163=AXIS2_PLACEMENT_3D ( 'NONE', #2398, #6730, #9607 ) ;
#11164=CYLINDRICAL_SURFACE ( 'NONE', #11876, 0.9999999999999991118 ) ;
#11166=DIRECTION ( 'NONE',  ( 0.000000000000000000, 0.000000000000000000, -1.000000000000000000 ) ) ;
#11169=CLOSED_SHELL ( 'NONE', ( #5225, #12379, #6480, #6610, #12582, #16360, #11186, #6545, #15031, #6432 ) ) ;
#11172=DIRECTION ( 'NONE',  ( -4.915049848600951133E-16, 0.000000000000000000, -1.000000000000000000 ) ) ;
#11179=EDGE_CURVE ( 'NONE', #8695, #2685, #9099, .T. ) ;
#11186=ADVANCED_FACE ( 'NONE', ( #15189 ), #1706, .T. ) ;
#11191=CIRCLE ( 'NONE', #4685, 0.9999999999999991118 ) ;
#11202=DIRECTION ( 'NONE',  ( 0.000000000000000000, 0.000000000000000000, -1.000000000000000000 ) ) ;
#11206=CIRCLE ( 'NONE', #12094, 0.9999999999999991118 ) ;
#11211=VERTEX_POINT ( 'NONE', #7178 ) ;
#11221=CARTESIAN_POINT ( 'NONE',  ( 9.000000000000001776, 40.79999999999999716, -2.500000000000002665 ) ) ;
#11222=EDGE_LOOP ( 'NONE', ( #10752, #11394, #2108, #13494 ) ) ;
#11225=EDGE_CURVE ( 'NONE', #1579, #15990, #11762, .T. ) ;
#11229=VERTEX_POINT ( 'NONE', #11083 ) ;
#11242=DIRECTION ( 'NONE',  ( -1.000000000000000000, 0.000000000000000000, 4.336808689942021680E-16 ) ) ;
#11243=ADVANCED_FACE ( 'NONE', ( #4228 ), #6437, .T. ) ;
#11252=CARTESIAN_POINT ( 'NONE',  ( -9.000000000000003553, 40.79999999999999716, -2.500000000000001776 ) ) ;
#11257=( LENGTH_UNIT ( ) NAMED_UNIT ( * ) SI_UNIT ( .MILLI., .METRE. ) );
#11266=AXIS2_PLACEMENT_3D ( 'NONE', #17513, #7460, #13024 ) ;
#11272=DIRECTION ( 'NONE',  ( -1.000000000000000000, 0.000000000000000000, 0.000000000000000000 ) ) ;
#11284=DIRECTION ( 'NONE',  ( 0.000000000000000000, 0.000000000000000000, -1.000000000000000000 ) ) ;
#11285=ORIENTED_EDGE ( 'NONE', *, *, #13407, .F. ) ;
#11299=CIRCLE ( 'NONE', #3330, 8.000000000000001776 ) ;
#11308=ORIENTED_EDGE ( 'NONE', *, *, #15246, .T. ) ;
#11314=DIRECTION ( 'NONE',  ( -0.000000000000000000, -1.000000000000000000, -0.000000000000000000 ) ) ;
#11322=CYLINDRICAL_SURFACE ( 'NONE', #8101, 0.9999999999999991118 ) ;
#11325=CIRCLE ( 'NONE', #11046, 10.00000000000000000 ) ;
#11327=CARTESIAN_POINT ( 'NONE',  ( -8.000000000000001776, 40.79999999999999716, 2.499999999999995115 ) ) ;
#11328=DIRECTION ( 'NONE',  ( 0.000000000000000000, 0.000000000000000000, -1.000000000000000000 ) ) ;
#11337=CARTESIAN_POINT ( 'NONE',  ( 8.000000000000000000, 31.99999999999999289, -2.500000000000000888 ) ) ;
#11338=DIRECTION ( 'NONE',  ( -1.000000000000000000, 0.000000000000000000, 0.000000000000000000 ) ) ;
#11341=CARTESIAN_POINT ( 'NONE',  ( -1.734723475976807094E-15, 20.99999999999999289, -2.500000000000000000 ) ) ;
#11350=DIRECTION ( 'NONE',  ( 0.000000000000000000, 0.000000000000000000, -1.000000000000000000 ) ) ;
#11352=ORIENTED_EDGE ( 'NONE', *, *, #17501, .F. ) ;
#11353=DIRECTION ( 'NONE',  ( -0.000000000000000000, -1.000000000000000000, -0.000000000000000000 ) ) ;
#11361=ORIENTED_EDGE ( 'NONE', *, *, #18236, .T. ) ;
#11366=AXIS2_PLACEMENT_3D ( 'NONE', #13590, #3949, #905 ) ;
#11372=ORIENTED_EDGE ( 'NONE', *, *, #8930, .F. ) ;
#11386=ORIENTED_EDGE ( 'NONE', *, *, #8030, .T. ) ;
#11394=ORIENTED_EDGE ( 'NONE', *, *, #2209, .T. ) ;
#11395=ORIENTED_EDGE ( 'NONE', *, *, #9827, .F. ) ;
#11397=CARTESIAN_POINT ( 'NONE',  ( -9.000000000000001776, 36.39999999999999147, 2.499999999999995559 ) ) ;
#11399=CARTESIAN_POINT ( 'NONE',  ( 10.00000000000000355, 18.79999999999999361, 2.499999999999996891 ) ) ;
#11416=CLOSED_SHELL ( 'NONE', ( #10432, #16185, #12324, #721, #14549, #225, #2214, #14493, #10933, #14552 ) ) ;
#11421=AXIS2_PLACEMENT_3D ( 'NONE', #907, #2219, #5342 ) ;
#11426=VERTEX_POINT ( 'NONE', #18254 ) ;
#11431=AXIS2_PLACEMENT_3D ( 'NONE', #8723, #13181, #1798 ) ;
#11444=CARTESIAN_POINT ( 'NONE',  ( 0.000000000000000000, 18.79999999999999361, 2.500000000000000000 ) ) ;
#11447=VECTOR ( 'NONE', #1653, 1000.000000000000000 ) ;
#11459=FACE_OUTER_BOUND ( 'NONE', #8691, .T. ) ;
#11461=EDGE_LOOP ( 'NONE', ( #14172, #10544, #14580, #4596 ) ) ;
#11465=ORIENTED_EDGE ( 'NONE', *, *, #14526, .F. ) ;
#11467=DIRECTION ( 'NONE',  ( -3.373073425510457965E-16, 0.000000000000000000, -1.000000000000000000 ) ) ;
#11488=ORIENTED_EDGE ( 'NONE', *, *, #3605, .F. ) ;
#11490=FACE_OUTER_BOUND ( 'NONE', #10014, .T. ) ;
#11491=CARTESIAN_POINT ( 'NONE',  ( 10.00000000000000355, 43.00000000000000000, 2.499999999999996891 ) ) ;
#11502=AXIS2_PLACEMENT_3D ( 'NONE', #12768, #7107, #15930 ) ;
#11510=CARTESIAN_POINT ( 'NONE',  ( -1.734723475976807094E-15, 29.79999999999999716, -2.500000000000000000 ) ) ;
#11514=DIRECTION ( 'NONE',  ( 3.469446951953612217E-16, -0.000000000000000000, 1.000000000000000000 ) ) ;
#11516=AXIS2_PLACEMENT_3D ( 'NONE', #908, #8305, #2758 ) ;
#11518=ADVANCED_FACE ( 'NONE', ( #13022 ), #9110, .T. ) ;
#11527=CIRCLE ( 'NONE', #15693, 0.9999999999999991118 ) ;
#11528=DIRECTION ( 'NONE',  ( 0.000000000000000000, 0.000000000000000000, -1.000000000000000000 ) ) ;
#11531=DIRECTION ( 'NONE',  ( 0.000000000000000000, 0.000000000000000000, -1.000000000000000000 ) ) ;
#11537=EDGE_CURVE ( 'NONE', #723, #1579, #13249, .T. ) ;
#11557=ORIENTED_EDGE ( 'NONE', *, *, #9600, .T. ) ;
#11571=EDGE_CURVE ( 'NONE', #9180, #4032, #9978, .T. ) ;
#11573=EDGE_CURVE ( 'NONE', #16267, #17729, #1432, .T. ) ;
#11576=EDGE_CURVE ( 'NONE', #9180, #7134, #5975, .T. ) ;
#11581=ORIENTED_EDGE ( 'NONE', *, *, #15525, .T. ) ;
#11584=CARTESIAN_POINT ( 'NONE',  ( -1.734723475976807094E-15, 16.59999999999999787, -10.50000000000000178 ) ) ;
#11593=CIRCLE ( 'NONE', #16958, 0.9999999999999991118 ) ;
#11600=CARTESIAN_POINT ( 'NONE',  ( 10.00000000000000000, 16.59999999999999787, -2.500000000000003109 ) ) ;
#11601=AXIS2_PLACEMENT_3D ( 'NONE', #11126, #18213, #5481 ) ;
#11604=DIRECTION ( 'NONE',  ( 0.000000000000000000, 0.000000000000000000, 1.000000000000000000 ) ) ;
#11607=ORIENTED_EDGE ( 'NONE', *, *, #9214, .F. ) ;
#11610=DIRECTION ( 'NONE',  ( 1.000000000000000000, 0.000000000000000000, -4.336808689942021680E-16 ) ) ;
#11611=VERTEX_POINT ( 'NONE', #8846 ) ;
#11620=AXIS2_PLACEMENT_3D ( 'NONE', #15871, #3075, #7139 ) ;
#11624=CARTESIAN_POINT ( 'NONE',  ( 8.000000000000000000, 40.79999999999999716, -2.500000000000000888 ) ) ;
#11631=TOROIDAL_SURFACE ( 'NONE', #7153, 9.000000000000003553, 0.9999999999999991118 ) ;
#11637=CARTESIAN_POINT ( 'NONE',  ( -1.734723475976807094E-15, 29.79999999999999716, -2.500000000000000000 ) ) ;
#11639=ORIENTED_EDGE ( 'NONE', *, *, #7933, .T. ) ;
#11668=VERTEX_POINT ( 'NONE', #3395 ) ;
#11674=DIRECTION ( 'NONE',  ( 0.000000000000000000, 0.000000000000000000, -1.000000000000000000 ) ) ;
#11683=EDGE_CURVE ( 'NONE', #1143, #1567, #7324, .T. ) ;
#11693=CARTESIAN_POINT ( 'NONE',  ( -10.00000000000000000, 36.39999999999999147, 2.499999999999998224 ) ) ;
#11698=ORIENTED_EDGE ( 'NONE', *, *, #14417, .T. ) ;
#11717=CARTESIAN_POINT ( 'NONE',  ( -8.000000000000003553, 43.00000000000000000, -2.500000000000001776 ) ) ;
#11719=AXIS2_PLACEMENT_3D ( 'NONE', #8747, #4676, #10325 ) ;
#11722=DIRECTION ( 'NONE',  ( -0.000000000000000000, -1.000000000000000000, -0.000000000000000000 ) ) ;
#11724=ORIENTED_EDGE ( 'NONE', *, *, #9701, .T. ) ;
#11734=ORIENTED_EDGE ( 'NONE', *, *, #2712, .T. ) ;
#11735=FACE_OUTER_BOUND ( 'NONE', #13316, .T. ) ;
#11743=EDGE_CURVE ( 'NONE', #3783, #1108, #17785, .T. ) ;
#11751=DIRECTION ( 'NONE',  ( -3.469446951953613696E-16, -0.000000000000000000, -1.000000000000000000 ) ) ;
#11762=CIRCLE ( 'NONE', #8495, 10.00000000000000000 ) ;
#11771=CARTESIAN_POINT ( 'NONE',  ( 9.000000000000005329, 43.00000000000000000, 2.499999999999997335 ) ) ;
#11773=DIRECTION ( 'NONE',  ( -0.000000000000000000, -1.000000000000000000, -0.000000000000000000 ) ) ;
#11778=AXIS2_PLACEMENT_3D ( 'NONE', #14713, #335, #10138 ) ;
#11785=LINE ( 'NONE', #14395, #11881 ) ;
#11787=EDGE_CURVE ( 'NONE', #15972, #6854, #8510, .T. ) ;
#11791=EDGE_LOOP ( 'NONE', ( #16143, #1439, #3464, #11285 ) ) ;
#11795=CARTESIAN_POINT ( 'NONE',  ( -1.734723475976807094E-15, 18.79999999999999361, -10.50000000000000178 ) ) ;
#11797=EDGE_LOOP ( 'NONE', ( #15557, #14694, #4362, #14403 ) ) ;
#11801=CIRCLE ( 'NONE', #573, 0.9999999999999991118 ) ;
#11802=DIRECTION ( 'NONE',  ( 0.000000000000000000, 0.000000000000000000, -1.000000000000000000 ) ) ;
#11818=DIRECTION ( 'NONE',  ( 1.000000000000000000, 0.000000000000000000, -4.336808689942021680E-16 ) ) ;
#11825=VECTOR ( 'NONE', #14314, 1000.000000000000000 ) ;
#11836=CARTESIAN_POINT ( 'NONE',  ( -8.000000000000001776, 27.59999999999999432, 2.499999999999998224 ) ) ;
#11843=AXIS2_PLACEMENT_3D ( 'NONE', #616, #2196, #11994 ) ;
#11844=DIRECTION ( 'NONE',  ( 0.000000000000000000, 0.000000000000000000, -1.000000000000000000 ) ) ;
#11852=EDGE_LOOP ( 'NONE', ( #1192, #2360, #10963, #2890 ) ) ;
#11859=ADVANCED_FACE ( 'NONE', ( #5328 ), #2470, .T. ) ;
#11865=ORIENTED_EDGE ( 'NONE', *, *, #2210, .F. ) ;
#11876=AXIS2_PLACEMENT_3D ( 'NONE', #15627, #4400, #8384 ) ;
#11881=VECTOR ( 'NONE', #14690, 1000.000000000000000 ) ;
#11884=LINE ( 'NONE', #12158, #2971 ) ;
#11888=DIRECTION ( 'NONE',  ( 0.000000000000000000, 0.000000000000000000, 1.000000000000000000 ) ) ;
#11903=CIRCLE ( 'NONE', #13083, 10.00000000000000000 ) ;
#11906=CARTESIAN_POINT ( 'NONE',  ( -1.734723475976807094E-15, 25.39999999999999503, -12.50000000000000000 ) ) ;
#11917=ADVANCED_FACE ( 'NONE', ( #9583 ), #793, .T. ) ;
#11924=EDGE_CURVE ( 'NONE', #8582, #894, #16235, .T. ) ;
#11926=VERTEX_POINT ( 'NONE', #15073 ) ;
#11928=DIRECTION ( 'NONE',  ( 0.000000000000000000, 0.000000000000000000, -1.000000000000000000 ) ) ;
#11932=AXIS2_PLACEMENT_3D ( 'NONE', #6897, #7233, #484 ) ;
#11934=AXIS2_PLACEMENT_3D ( 'NONE', #6852, #5282, #11110 ) ;
#11938=EDGE_LOOP ( 'NONE', ( #12714, #14127, #9109, #9641 ) ) ;
#11943=ORIENTED_EDGE ( 'NONE', *, *, #85, .F. ) ;
#11946=FACE_OUTER_BOUND ( 'NONE', #11049, .T. ) ;
#11957=DIRECTION ( 'NONE',  ( 3.469446951953612217E-16, -0.000000000000000000, 1.000000000000000000 ) ) ;
#11960=AXIS2_PLACEMENT_3D ( 'NONE', #5696, #13010, #5781 ) ;
#11962=ORIENTED_EDGE ( 'NONE', *, *, #15229, .F. ) ;
#11964=DIRECTION ( 'NONE',  ( -0.000000000000000000, -1.000000000000000000, -0.000000000000000000 ) ) ;
#11978=CARTESIAN_POINT ( 'NONE',  ( -1.734723475976807094E-15, 40.79999999999999716, -2.500000000000000000 ) ) ;
#11982=CARTESIAN_POINT ( 'NONE',  ( 8.000000000000005329, 43.00000000000000000, 2.499999999999997780 ) ) ;
#11983=CARTESIAN_POINT ( 'NONE',  ( 10.00000000000000000, 20.99999999999999289, -2.500000000000003109 ) ) ;
#11994=DIRECTION ( 'NONE',  ( 0.000000000000000000, 0.000000000000000000, -1.000000000000000000 ) ) ;
#11998=EDGE_LOOP ( 'NONE', ( #4296, #1658, #3140, #1353 ) ) ;
#11999=FACE_OUTER_BOUND ( 'NONE', #9383, .T. ) ;
#12007=VERTEX_POINT ( 'NONE', #7157 ) ;
#12012=TOROIDAL_SURFACE ( 'NONE', #9353, 9.000000000000001776, 0.9999999999999991118 ) ;
#12015=DIRECTION ( 'NONE',  ( -0.000000000000000000, -1.000000000000000000, -0.000000000000000000 ) ) ;
#12018=CARTESIAN_POINT ( 'NONE',  ( -1.734723475976807094E-15, 16.59999999999999787, -11.50000000000000178 ) ) ;
#12025=ORIENTED_EDGE ( 'NONE', *, *, #9598, .T. ) ;
#12027=CARTESIAN_POINT ( 'NONE',  ( -1.734723475976807094E-15, 43.00000000000000000, -2.500000000000000000 ) ) ;
#12054=CARTESIAN_POINT ( 'NONE',  ( -1.734723475976807094E-15, 31.99999999999999289, -11.50000000000000178 ) ) ;
#12066=ORIENTED_EDGE ( 'NONE', *, *, #6323, .T. ) ;
#12080=TOROIDAL_SURFACE ( 'NONE', #4087, 9.000000000000001776, 0.9999999999999991118 ) ;
#12082=TOROIDAL_SURFACE ( 'NONE', #17453, 9.000000000000001776, 0.9999999999999991118 ) ;
#12085=DIRECTION ( 'NONE',  ( 0.000000000000000000, 0.000000000000000000, 1.000000000000000000 ) ) ;
#12086=ADVANCED_FACE ( 'NONE', ( #1436 ), #12082, .T. ) ;
#12094=AXIS2_PLACEMENT_3D ( 'NONE', #3162, #8799, #3258 ) ;
#12095=ORIENTED_EDGE ( 'NONE', *, *, #6327, .F. ) ;
#12105=CARTESIAN_POINT ( 'NONE',  ( -9.000000000000001776, 29.79999999999999716, 2.499999999999998224 ) ) ;
#12108=DIRECTION ( 'NONE',  ( -3.469446951953613696E-16, -0.000000000000000000, -1.000000000000000000 ) ) ;
#12114=CARTESIAN_POINT ( 'NONE',  ( 8.000000000000001776, 34.19999999999999574, -2.500000000000002220 ) ) ;
#12121=AXIS2_PLACEMENT_3D ( 'NONE', #18190, #8494, #17059 ) ;
#12129=DIRECTION ( 'NONE',  ( 0.000000000000000000, 0.000000000000000000, -1.000000000000000000 ) ) ;
#12132=CIRCLE ( 'NONE', #7096, 8.000000000000001776 ) ;
#12136=EDGE_LOOP ( 'NONE', ( #1242, #4915, #2325, #10946 ) ) ;
#12143=DIRECTION ( 'NONE',  ( 0.000000000000000000, 0.000000000000000000, 1.000000000000000000 ) ) ;
#12149=ADVANCED_FACE ( 'NONE', ( #6803 ), #13276, .T. ) ;
#12158=CARTESIAN_POINT ( 'NONE',  ( 8.000000000000001776, 40.79999999999999716, -2.500000000000002220 ) ) ;
#12160=ORIENTED_EDGE ( 'NONE', *, *, #2798, .F. ) ;
#12163=EDGE_CURVE ( 'NONE', #3667, #723, #10908, .T. ) ;
#12165=CARTESIAN_POINT ( 'NONE',  ( 8.000000000000001776, 27.59999999999999432, -2.500000000000002220 ) ) ;
#12174=CIRCLE ( 'NONE', #5154, 0.9999999999999991118 ) ;
#12179=DIRECTION ( 'NONE',  ( -1.000000000000000000, 0.000000000000000000, 0.000000000000000000 ) ) ;
#12183=DIRECTION ( 'NONE',  ( -3.469446951953613696E-16, -0.000000000000000000, -1.000000000000000000 ) ) ;
#12190=CYLINDRICAL_SURFACE ( 'NONE', #686, 0.9999999999999991118 ) ;
#12192=ORIENTED_EDGE ( 'NONE', *, *, #4453, .T. ) ;
#12196=ORIENTED_EDGE ( 'NONE', *, *, #6323, .F. ) ;
#12200=DIRECTION ( 'NONE',  ( -0.000000000000000000, -1.000000000000000000, -0.000000000000000000 ) ) ;
#12216=ORIENTED_EDGE ( 'NONE', *, *, #9827, .T. ) ;
#12218=ADVANCED_FACE ( 'NONE', ( #17486 ), #7616, .T. ) ;
#12221=TOROIDAL_SURFACE ( 'NONE', #4232, 9.000000000000001776, 0.9999999999999991118 ) ;
#12241=ORIENTED_EDGE ( 'NONE', *, *, #9556, .T. ) ;
#12251=FACE_OUTER_BOUND ( 'NONE', #9323, .T. ) ;
#12253=VERTEX_POINT ( 'NONE', #7244 ) ;
#12269=DIRECTION ( 'NONE',  ( 3.469446951953612217E-16, -0.000000000000000000, 1.000000000000000000 ) ) ;
#12277=DIRECTION ( 'NONE',  ( -1.000000000000000000, 0.000000000000000000, 4.336808689942021680E-16 ) ) ;
#12288=EDGE_CURVE ( 'NONE', #8695, #1204, #9123, .T. ) ;
#12290=CARTESIAN_POINT ( 'NONE',  ( -1.734723475976807094E-15, 29.79999999999999716, -10.50000000000000178 ) ) ;
#12295=CARTESIAN_POINT ( 'NONE',  ( 9.000000000000005329, 36.39999999999999147, 2.499999999999997335 ) ) ;
#12298=VERTEX_POINT ( 'NONE', #6237 ) ;
#12299=ORIENTED_EDGE ( 'NONE', *, *, #7385, .F. ) ;
#12300=CARTESIAN_POINT ( 'NONE',  ( 0.000000000000000000, 34.19999999999999574, 2.500000000000000000 ) ) ;
#12304=AXIS2_PLACEMENT_3D ( 'NONE', #11060, #11145, #13940 ) ;
#12305=ORIENTED_EDGE ( 'NONE', *, *, #8930, .T. ) ;
#12317=EDGE_CURVE ( 'NONE', #13188, #9609, #7044, .T. ) ;
#12318=CARTESIAN_POINT ( 'NONE',  ( -8.000000000000001776, 18.79999999999999361, 2.499999999999995115 ) ) ;
#12324=ADVANCED_FACE ( 'NONE', ( #4655 ), #3507, .T. ) ;
#12340=DIRECTION ( 'NONE',  ( 1.000000000000000000, 0.000000000000000000, 0.000000000000000000 ) ) ;
#12343=LINE ( 'NONE', #8173, #12973 ) ;
#12347=VERTEX_POINT ( 'NONE', #14398 ) ;
#12349=AXIS2_PLACEMENT_3D ( 'NONE', #13876, #18074, #8211 ) ;
#12353=CARTESIAN_POINT ( 'NONE',  ( 9.000000000000001776, 40.79999999999999716, -2.500000000000002665 ) ) ;
#12355=EDGE_CURVE ( 'NONE', #9649, #2406, #9419, .T. ) ;
#12356=AXIS2_PLACEMENT_3D ( 'NONE', #15657, #266, #1852 ) ;
#12357=AXIS2_PLACEMENT_3D ( 'NONE', #9222, #6353, #13480 ) ;
#12368=AXIS2_PLACEMENT_3D ( 'NONE', #15268, #15080, #5423 ) ;
#12371=CARTESIAN_POINT ( 'NONE',  ( 9.000000000000001776, 18.79999999999999361, -2.500000000000002665 ) ) ;
#12374=VERTEX_POINT ( 'NONE', #2267 ) ;
#12378=EDGE_CURVE ( 'NONE', #13359, #12413, #565, .T. ) ;
#12379=ADVANCED_FACE ( 'NONE', ( #13739 ), #2920, .T. ) ;
#12380=DIRECTION ( 'NONE',  ( -0.000000000000000000, -1.000000000000000000, -0.000000000000000000 ) ) ;
#12383=CARTESIAN_POINT ( 'NONE',  ( -8.000000000000001776, 16.59999999999999787, 2.499999999999995115 ) ) ;
#12393=ORIENTED_EDGE ( 'NONE', *, *, #3325, .T. ) ;
#12401=CIRCLE ( 'NONE', #4403, 0.9999999999999991118 ) ;
#12411=VECTOR ( 'NONE', #9606, 1000.000000000000000 ) ;
#12413=VERTEX_POINT ( 'NONE', #14970 ) ;
#12433=DIRECTION ( 'NONE',  ( 3.469446951953612217E-16, -0.000000000000000000, 1.000000000000000000 ) ) ;
#12435=DIRECTION ( 'NONE',  ( 0.000000000000000000, 0.000000000000000000, -1.000000000000000000 ) ) ;
#12437=ORIENTED_EDGE ( 'NONE', *, *, #15775, .F. ) ;
#12440=CYLINDRICAL_SURFACE ( 'NONE', #5676, 0.9999999999999991118 ) ;
#12443=VECTOR ( 'NONE', #15887, 1000.000000000000000 ) ;
#12448=CARTESIAN_POINT ( 'NONE',  ( 8.000000000000000000, 34.19999999999999574, -2.500000000000000888 ) ) ;
#12458=DIRECTION ( 'NONE',  ( -3.469446951953613696E-16, -0.000000000000000000, -1.000000000000000000 ) ) ;
#12462=CARTESIAN_POINT ( 'NONE',  ( -1.734723475976807094E-15, 43.00000000000000000, -2.500000000000000000 ) ) ;
#12467=CARTESIAN_POINT ( 'NONE',  ( 0.000000000000000000, 25.39999999999999503, 2.500000000000000000 ) ) ;
#12469=DIRECTION ( 'NONE',  ( -0.000000000000000000, -1.000000000000000000, -0.000000000000000000 ) ) ;
#12471=ADVANCED_FACE ( 'NONE', ( #13372 ), #2908, .T. ) ;
#12472=ORIENTED_EDGE ( 'NONE', *, *, #4423, .F. ) ;
#12479=CIRCLE ( 'NONE', #5088, 10.00000000000000178 ) ;
#12482=UNCERTAINTY_MEASURE_WITH_UNIT (LENGTH_MEASURE( 1.000000000000000082E-05 ), #443, 'distance_accuracy_value', 'NONE');
#12484=DIRECTION ( 'NONE',  ( 0.000000000000000000, 0.000000000000000000, -1.000000000000000000 ) ) ;
#12486=EDGE_LOOP ( 'NONE', ( #8171, #2038, #11133, #6490 ) ) ;
#12488=EDGE_CURVE ( 'NONE', #11229, #12007, #18033, .T. ) ;
#12500=ORIENTED_EDGE ( 'NONE', *, *, #15796, .T. ) ;
#12501=CYLINDRICAL_SURFACE ( 'NONE', #18345, 0.9999999999999991118 ) ;
#12505=DIRECTION ( 'NONE',  ( -3.373073425510457965E-16, 0.000000000000000000, -1.000000000000000000 ) ) ;
#12513=CIRCLE ( 'NONE', #12814, 0.9999999999999991118 ) ;
#12523=EDGE_CURVE ( 'NONE', #13188, #11611, #11191, .T. ) ;
#12527=DIRECTION ( 'NONE',  ( 0.000000000000000000, 0.000000000000000000, -1.000000000000000000 ) ) ;
#12529=ORIENTED_EDGE ( 'NONE', *, *, #4221, .F. ) ;
#12534=ORIENTED_EDGE ( 'NONE', *, *, #6901, .F. ) ;
#12539=DIRECTION ( 'NONE',  ( -0.000000000000000000, -1.000000000000000000, -0.000000000000000000 ) ) ;
#12543=DIRECTION ( 'NONE',  ( -1.000000000000000000, 0.000000000000000000, 4.336808689942021680E-16 ) ) ;
#12544=ADVANCED_FACE ( 'NONE', ( #9377 ), #15053, .T. ) ;
#12553=ADVANCED_FACE ( 'NONE', ( #12251 ), #3817, .T. ) ;
#12559=CIRCLE ( 'NONE', #13452, 0.9999999999999991118 ) ;
#12563=CARTESIAN_POINT ( 'NONE',  ( 9.000000000000000000, 36.39999999999999147, -2.500000000000001332 ) ) ;
#12569=CARTESIAN_POINT ( 'NONE',  ( -10.00000000000000000, 23.19999999999999574, 2.499999999999998224 ) ) ;
#12582=ADVANCED_FACE ( 'NONE', ( #1235 ), #1413, .T. ) ;
#12601=ORIENTED_EDGE ( 'NONE', *, *, #6638, .F. ) ;
#12613=DIRECTION ( 'NONE',  ( -0.000000000000000000, -1.000000000000000000, -0.000000000000000000 ) ) ;
#12614=DIRECTION ( 'NONE',  ( -0.000000000000000000, -1.000000000000000000, -0.000000000000000000 ) ) ;
#12622=VERTEX_POINT ( 'NONE', #5485 ) ;
#12628=AXIS2_PLACEMENT_3D ( 'NONE', #13114, #426, #3206 ) ;
#12629=DIRECTION ( 'NONE',  ( 0.000000000000000000, 0.000000000000000000, 1.000000000000000000 ) ) ;
#12633=ADVANCED_FACE ( 'NONE', ( #8353 ), #13865, .T. ) ;
#12652=CARTESIAN_POINT ( 'NONE',  ( 8.000000000000005329, 34.19999999999999574, 2.499999999999997780 ) ) ;
#12653=EDGE_CURVE ( 'NONE', #9649, #17767, #7644, .T. ) ;
#12657=ORIENTED_EDGE ( 'NONE', *, *, #16764, .F. ) ;
#12658=DIRECTION ( 'NONE',  ( 0.000000000000000000, 0.000000000000000000, -1.000000000000000000 ) ) ;
#12664=CARTESIAN_POINT ( 'NONE',  ( -10.00000000000000000, 38.59999999999999432, 2.499999999999998224 ) ) ;
#12671=VECTOR ( 'NONE', #6808, 1000.000000000000000 ) ;
#12678=( NAMED_UNIT ( * ) SI_UNIT ( $, .STERADIAN. ) SOLID_ANGLE_UNIT ( ) );
#12680=DIRECTION ( 'NONE',  ( -0.000000000000000000, -1.000000000000000000, -0.000000000000000000 ) ) ;
#12682=EDGE_LOOP ( 'NONE', ( #13730, #9706, #7760, #11465 ) ) ;
#12683=FACE_OUTER_BOUND ( 'NONE', #10091, .T. ) ;
#12690=TOROIDAL_SURFACE ( 'NONE', #15372, 9.000000000000001776, 0.9999999999999991118 ) ;
#12696=ORIENTED_EDGE ( 'NONE', *, *, #4861, .T. ) ;
#12700=AXIS2_PLACEMENT_3D ( 'NONE', #6185, #16303, #17624 ) ;
#12702=AXIS2_PLACEMENT_3D ( 'NONE', #10654, #3251, #17362 ) ;
#12714=ORIENTED_EDGE ( 'NONE', *, *, #2483, .F. ) ;
#12720=EDGE_CURVE ( 'NONE', #17541, #15647, #15920, .T. ) ;
#12723=DIRECTION ( 'NONE',  ( -0.000000000000000000, -1.000000000000000000, -0.000000000000000000 ) ) ;
#12726=EDGE_CURVE ( 'NONE', #2412, #18202, #14434, .T. ) ;
#12728=EDGE_CURVE ( 'NONE', #14997, #13741, #4995, .T. ) ;
#12732=AXIS2_PLACEMENT_3D ( 'NONE', #5900, #4328, #71 ) ;
#12747=DIRECTION ( 'NONE',  ( 0.000000000000000000, 0.000000000000000000, -1.000000000000000000 ) ) ;
#12750=LINE ( 'NONE', #5343, #6199 ) ;
#12760=DIRECTION ( 'NONE',  ( -3.469446951953613696E-16, -0.000000000000000000, -1.000000000000000000 ) ) ;
#12766=VECTOR ( 'NONE', #4470, 1000.000000000000000 ) ;
#12768=CARTESIAN_POINT ( 'NONE',  ( 9.000000000000005329, 38.59999999999999432, 2.499999999999997335 ) ) ;
#12776=EDGE_LOOP ( 'NONE', ( #1734, #16796, #10074, #10372 ) ) ;
#12786=VERTEX_POINT ( 'NONE', #17462 ) ;
#12796=FACE_OUTER_BOUND ( 'NONE', #1104, .T. ) ;
#12813=EDGE_CURVE ( 'NONE', #18266, #156, #15649, .T. ) ;
#12814=AXIS2_PLACEMENT_3D ( 'NONE', #9007, #6224, #2345 ) ;
#12815=AXIS2_PLACEMENT_3D ( 'NONE', #9836, #15776, #17089 ) ;
#12818=CARTESIAN_POINT ( 'NONE',  ( -1.734723475976807094E-15, 36.39999999999999147, -11.50000000000000178 ) ) ;
#12826=AXIS2_PLACEMENT_3D ( 'NONE', #17234, #14155, #8760 ) ;
#12836=DIRECTION ( 'NONE',  ( -1.000000000000000000, 0.000000000000000000, 4.336808689942021680E-16 ) ) ;
#12837=TOROIDAL_SURFACE ( 'NONE', #1647, 9.000000000000001776, 0.9999999999999991118 ) ;
#12839=CARTESIAN_POINT ( 'NONE',  ( -1.734723475976807094E-15, 27.59999999999999432, -2.500000000000000000 ) ) ;
#12860=ORIENTED_EDGE ( 'NONE', *, *, #11743, .F. ) ;
#12874=ADVANCED_FACE ( 'NONE', ( #12796 ), #255, .T. ) ;
#12887=CARTESIAN_POINT ( 'NONE',  ( -1.734723475976807094E-15, 16.59999999999999787, -2.500000000000000000 ) ) ;
#12888=CARTESIAN_POINT ( 'NONE',  ( -1.734723475976807094E-15, 27.59999999999999432, -2.500000000000000000 ) ) ;
#12889=EDGE_LOOP ( 'NONE', ( #6912, #5821, #7116, #8226 ) ) ;
#12897=AXIS2_PLACEMENT_3D ( 'NONE', #8357, #2632, #8083 ) ;
#12899=CIRCLE ( 'NONE', #175, 0.9999999999999991118 ) ;
#12901=DIRECTION ( 'NONE',  ( -0.000000000000000000, -1.000000000000000000, -0.000000000000000000 ) ) ;
#12909=AXIS2_PLACEMENT_3D ( 'NONE', #8470, #14140, #7084 ) ;
#12911=DIRECTION ( 'NONE',  ( -1.000000000000000000, 0.000000000000000000, 4.336808689942021680E-16 ) ) ;
#12912=FACE_OUTER_BOUND ( 'NONE', #3513, .T. ) ;
#12914=ADVANCED_FACE ( 'NONE', ( #1970 ), #12690, .T. ) ;
#12920=CIRCLE ( 'NONE', #8468, 0.9999999999999991118 ) ;
#12932=EDGE_CURVE ( 'NONE', #5635, #2806, #862, .T. ) ;
#12935=EDGE_CURVE ( 'NONE', #1567, #1143, #11206, .T. ) ;
#12936=AXIS2_PLACEMENT_3D ( 'NONE', #8567, #3022, #11350 ) ;
#12948=TOROIDAL_SURFACE ( 'NONE', #12356, 9.000000000000001776, 0.9999999999999991118 ) ;
#12956=DIRECTION ( 'NONE',  ( 0.000000000000000000, 0.000000000000000000, -1.000000000000000000 ) ) ;
#12957=DIRECTION ( 'NONE',  ( -3.469446951953613696E-16, -0.000000000000000000, -1.000000000000000000 ) ) ;
#12965=AXIS2_PLACEMENT_3D ( 'NONE', #4540, #3064, #16992 ) ;
#12973=VECTOR ( 'NONE', #17850, 1000.000000000000000 ) ;
#12976=AXIS2_PLACEMENT_3D ( 'NONE', #1680, #5932, #8609 ) ;
#12990=LINE ( 'NONE', #304, #14079 ) ;
#13004=ORIENTED_EDGE ( 'NONE', *, *, #6249, .T. ) ;
#13010=DIRECTION ( 'NONE',  ( -0.000000000000000000, -1.000000000000000000, -0.000000000000000000 ) ) ;
#13022=FACE_OUTER_BOUND ( 'NONE', #1499, .T. ) ;
#13024=DIRECTION ( 'NONE',  ( -1.000000000000000000, 0.000000000000000000, 4.336808689942021680E-16 ) ) ;
#13029=DIRECTION ( 'NONE',  ( -3.373073425510457965E-16, 0.000000000000000000, -1.000000000000000000 ) ) ;
#13031=AXIS2_PLACEMENT_3D ( 'NONE', #16264, #3553, #4753 ) ;
#13032=DIRECTION ( 'NONE',  ( -0.000000000000000000, -1.000000000000000000, -0.000000000000000000 ) ) ;
#13034=EDGE_LOOP ( 'NONE', ( #738, #7994, #6196, #8703 ) ) ;
#13039=EDGE_CURVE ( 'NONE', #6854, #15972, #4394, .T. ) ;
#13042=AXIS2_PLACEMENT_3D ( 'NONE', #5527, #9960, #2582 ) ;
#13049=ADVANCED_FACE ( 'NONE', ( #6215 ), #3523, .T. ) ;
#13054=DIRECTION ( 'NONE',  ( 1.000000000000000000, 0.000000000000000000, 0.000000000000000000 ) ) ;
#13068=AXIS2_PLACEMENT_3D ( 'NONE', #2362, #5490, #7991 ) ;
#13075=CARTESIAN_POINT ( 'NONE',  ( 9.000000000000005329, 34.19999999999999574, 2.499999999999997335 ) ) ;
#13083=AXIS2_PLACEMENT_3D ( 'NONE', #16914, #17187, #15688 ) ;
#13090=CARTESIAN_POINT ( 'NONE',  ( -1.734723475976807094E-15, 34.19999999999999574, -2.500000000000000000 ) ) ;
#13092=CIRCLE ( 'NONE', #5702, 0.9999999999999991118 ) ;
#13114=CARTESIAN_POINT ( 'NONE',  ( -1.734723475976807094E-15, 18.79999999999999361, -2.500000000000000000 ) ) ;
#13115=EDGE_CURVE ( 'NONE', #5913, #17692, #9134, .T. ) ;
#13118=CARTESIAN_POINT ( 'NONE',  ( -8.000000000000001776, 27.59999999999999432, 2.499999999999995115 ) ) ;
#13134=CARTESIAN_POINT ( 'NONE',  ( -9.000000000000001776, 34.19999999999999574, 2.499999999999995559 ) ) ;
#13135=CARTESIAN_POINT ( 'NONE',  ( 0.000000000000000000, 40.79999999999999716, 2.500000000000000000 ) ) ;
#13141=ORIENTED_EDGE ( 'NONE', *, *, #14785, .T. ) ;
#13143=CARTESIAN_POINT ( 'NONE',  ( -1.734723475976807094E-15, 40.79999999999999716, -12.50000000000000000 ) ) ;
#13144=FACE_OUTER_BOUND ( 'NONE', #5259, .T. ) ;
#13148=CARTESIAN_POINT ( 'NONE',  ( -8.000000000000001776, 31.99999999999999289, 2.499999999999995115 ) ) ;
#13155=ORIENTED_EDGE ( 'NONE', *, *, #6880, .T. ) ;
#13156=ADVANCED_FACE ( 'NONE', ( #15216 ), #12501, .T. ) ;
#13170=DIRECTION ( 'NONE',  ( 0.000000000000000000, 0.000000000000000000, 1.000000000000000000 ) ) ;
#13173=EDGE_CURVE ( 'NONE', #17672, #13234, #10317, .T. ) ;
#13174=EDGE_CURVE ( 'NONE', #2685, #3667, #4163, .T. ) ;
#13181=DIRECTION ( 'NONE',  ( 0.000000000000000000, 0.000000000000000000, 1.000000000000000000 ) ) ;
#13182=DIRECTION ( 'NONE',  ( 3.469446951953612217E-16, -0.000000000000000000, 1.000000000000000000 ) ) ;
#13183=DIRECTION ( 'NONE',  ( -1.000000000000000000, 0.000000000000000000, 4.336808689942021680E-16 ) ) ;
#13184=ORIENTED_EDGE ( 'NONE', *, *, #12653, .F. ) ;
#13187=CARTESIAN_POINT ( 'NONE',  ( -1.734723475976807094E-15, 16.59999999999999787, -2.500000000000000000 ) ) ;
#13188=VERTEX_POINT ( 'NONE', #18008 ) ;
#13197=EDGE_LOOP ( 'NONE', ( #15548, #12241, #6447, #12657 ) ) ;
#13198=DIRECTION ( 'NONE',  ( 0.000000000000000000, 0.000000000000000000, -1.000000000000000000 ) ) ;
#13206=DIRECTION ( 'NONE',  ( -3.469446951953613696E-16, -0.000000000000000000, -1.000000000000000000 ) ) ;
#13222=EDGE_CURVE ( 'NONE', #4161, #2412, #8253, .T. ) ;
#13227=DIRECTION ( 'NONE',  ( 0.000000000000000000, 0.000000000000000000, -1.000000000000000000 ) ) ;
#13234=VERTEX_POINT ( 'NONE', #16704 ) ;
#13235=CIRCLE ( 'NONE', #5245, 0.9999999999999991118 ) ;
#13236=ORIENTED_EDGE ( 'NONE', *, *, #15717, .T. ) ;
#13249=CIRCLE ( 'NONE', #3788, 10.00000000000000000 ) ;
#13254=TOROIDAL_SURFACE ( 'NONE', #7333, 9.000000000000001776, 0.9999999999999991118 ) ;
#13256=ORIENTED_EDGE ( 'NONE', *, *, #15796, .F. ) ;
#13258=DIRECTION ( 'NONE',  ( -1.000000000000000000, 0.000000000000000000, 4.336808689942021680E-16 ) ) ;
#13266=AXIS2_PLACEMENT_3D ( 'NONE', #16446, #7714, #2084 ) ;
#13272=CIRCLE ( 'NONE', #1464, 10.00000000000000000 ) ;
#13276=TOROIDAL_SURFACE ( 'NONE', #10605, 9.000000000000003553, 0.9999999999999991118 ) ;
#13279=CARTESIAN_POINT ( 'NONE',  ( -1.734723475976807094E-15, 43.00000000000000000, -2.500000000000000000 ) ) ;
#13280=ADVANCED_FACE ( 'NONE', ( #12683 ), #5544, .T. ) ;
#13281=DIRECTION ( 'NONE',  ( 0.000000000000000000, 0.000000000000000000, 1.000000000000000000 ) ) ;
#13288=EDGE_CURVE ( 'NONE', #6366, #17369, #1303, .T. ) ;
#13294=EDGE_CURVE ( 'NONE', #14197, #9655, #5560, .T. ) ;
#13299=TOROIDAL_SURFACE ( 'NONE', #15673, 9.000000000000003553, 0.9999999999999991118 ) ;
#13303=AXIS2_PLACEMENT_3D ( 'NONE', #4331, #14071, #5639 ) ;
#13308=CARTESIAN_POINT ( 'NONE',  ( -1.734723475976807094E-15, 20.99999999999999289, -2.500000000000000000 ) ) ;
#13314=CARTESIAN_POINT ( 'NONE',  ( -8.000000000000001776, 31.99999999999999289, 2.499999999999998224 ) ) ;
#13316=EDGE_LOOP ( 'NONE', ( #2359, #16549, #3223, #9185 ) ) ;
#13333=CIRCLE ( 'NONE', #2694, 0.9999999999999991118 ) ;
#13337=LINE ( 'NONE', #3335, #16971 ) ;
#13346=ORIENTED_EDGE ( 'NONE', *, *, #13976, .T. ) ;
#13347=TOROIDAL_SURFACE ( 'NONE', #6827, 9.000000000000003553, 0.9999999999999991118 ) ;
#13359=VERTEX_POINT ( 'NONE', #17253 ) ;
#13369=EDGE_CURVE ( 'NONE', #894, #2439, #1478, .T. ) ;
#13372=FACE_OUTER_BOUND ( 'NONE', #16406, .T. ) ;
#13376=AXIS2_PLACEMENT_3D ( 'NONE', #11397, #14292, #14381 ) ;
#13377=FACE_OUTER_BOUND ( 'NONE', #7207, .T. ) ;
#13396=ORIENTED_EDGE ( 'NONE', *, *, #17754, .F. ) ;
#13397=DIRECTION ( 'NONE',  ( -0.000000000000000000, -1.000000000000000000, -0.000000000000000000 ) ) ;
#13398=LINE ( 'NONE', #2202, #5893 ) ;
#13403=AXIS2_PLACEMENT_3D ( 'NONE', #15783, #17286, #13170 ) ;
#13407=EDGE_CURVE ( 'NONE', #13486, #1006, #7390, .T. ) ;
#13414=LINE ( 'NONE', #12383, #7886 ) ;
#13415=CARTESIAN_POINT ( 'NONE',  ( -1.734723475976807094E-15, 25.39999999999999503, -2.500000000000000000 ) ) ;
#13416=CIRCLE ( 'NONE', #5426, 0.9999999999999991118 ) ;
#13421=ORIENTED_EDGE ( 'NONE', *, *, #7103, .T. ) ;
#13427=( LENGTH_UNIT ( ) NAMED_UNIT ( * ) SI_UNIT ( .MILLI., .METRE. ) );
#13428=SURFACE_STYLE_FILL_AREA ( #7768 ) ;
#13432=CIRCLE ( 'NONE', #15806, 0.9999999999999991118 ) ;
#13439=DIRECTION ( 'NONE',  ( -1.000000000000000000, 0.000000000000000000, 4.336808689942021680E-16 ) ) ;
#13451=DIRECTION ( 'NONE',  ( -3.469446951953613696E-16, -0.000000000000000000, -1.000000000000000000 ) ) ;
#13452=AXIS2_PLACEMENT_3D ( 'NONE', #17736, #469, #13439 ) ;
#13458=ADVANCED_FACE ( 'NONE', ( #14265 ), #12948, .T. ) ;
#13466=ORIENTED_EDGE ( 'NONE', *, *, #9208, .F. ) ;
#13467=CARTESIAN_POINT ( 'NONE',  ( -1.734723475976807094E-15, 23.19999999999999574, -11.50000000000000178 ) ) ;
#13468=DIRECTION ( 'NONE',  ( 3.469446951953612217E-16, -0.000000000000000000, 1.000000000000000000 ) ) ;
#13480=DIRECTION ( 'NONE',  ( 1.000000000000000000, 0.000000000000000000, 0.000000000000000000 ) ) ;
#13483=DIRECTION ( 'NONE',  ( 0.000000000000000000, 0.000000000000000000, -1.000000000000000000 ) ) ;
#13486=VERTEX_POINT ( 'NONE', #7486 ) ;
#13494=ORIENTED_EDGE ( 'NONE', *, *, #9321, .F. ) ;
#13497=AXIS2_PLACEMENT_3D ( 'NONE', #9028, #7630, #2190 ) ;
#13498=DIRECTION ( 'NONE',  ( -3.469446951953613696E-16, -0.000000000000000000, -1.000000000000000000 ) ) ;
#13500=CARTESIAN_POINT ( 'NONE',  ( 9.000000000000005329, 40.79999999999999716, 2.499999999999997335 ) ) ;
#13503=ADVANCED_FACE ( 'NONE', ( #13144 ), #4526, .T. ) ;
#13508=ADVANCED_FACE ( 'NONE', ( #1569 ), #10167, .T. ) ;
#13517=EDGE_LOOP ( 'NONE', ( #17249, #9238, #6768, #17540 ) ) ;
#13521=VERTEX_POINT ( 'NONE', #6002 ) ;
#13522=CARTESIAN_POINT ( 'NONE',  ( -8.000000000000003553, 27.59999999999999432, -2.500000000000001776 ) ) ;
#13525=CARTESIAN_POINT ( 'NONE',  ( -9.000000000000001776, 36.39999999999999147, 2.499999999999998224 ) ) ;
#13530=ORIENTED_EDGE ( 'NONE', *, *, #9326, .T. ) ;
#13534=VERTEX_POINT ( 'NONE', #10982 ) ;
#13543=EDGE_LOOP ( 'NONE', ( #3677, #4705, #14647, #1554 ) ) ;
#13546=DIRECTION ( 'NONE',  ( -0.000000000000000000, -1.000000000000000000, -0.000000000000000000 ) ) ;
#13548=DIRECTION ( 'NONE',  ( -0.000000000000000000, -1.000000000000000000, -0.000000000000000000 ) ) ;
#13553=DIRECTION ( 'NONE',  ( 1.000000000000000000, 0.000000000000000000, -4.336808689942021680E-16 ) ) ;
#13555=ORIENTED_EDGE ( 'NONE', *, *, #13115, .T. ) ;
#13557=DIRECTION ( 'NONE',  ( 0.000000000000000000, 0.000000000000000000, 1.000000000000000000 ) ) ;
#13568=DIRECTION ( 'NONE',  ( 3.469446951953612217E-16, -0.000000000000000000, 1.000000000000000000 ) ) ;
#13570=ORIENTED_EDGE ( 'NONE', *, *, #17545, .F. ) ;
#13572=DIRECTION ( 'NONE',  ( -3.469446951953613696E-16, -0.000000000000000000, -1.000000000000000000 ) ) ;
#13575=EDGE_CURVE ( 'NONE', #634, #3783, #14756, .T. ) ;
#13576=AXIS2_PLACEMENT_3D ( 'NONE', #9450, #15123, #3706 ) ;
#13579=CARTESIAN_POINT ( 'NONE',  ( 0.000000000000000000, 36.39999999999999147, 2.500000000000000000 ) ) ;
#13581=DIRECTION ( 'NONE',  ( 0.000000000000000000, 0.000000000000000000, -1.000000000000000000 ) ) ;
#13587=AXIS2_PLACEMENT_3D ( 'NONE', #13308, #11722, #6260 ) ;
#13589=AXIS2_PLACEMENT_3D ( 'NONE', #15650, #1840, #4516 ) ;
#13590=CARTESIAN_POINT ( 'NONE',  ( -9.000000000000003553, 27.59999999999999432, -2.500000000000001776 ) ) ;
#13591=AXIS2_PLACEMENT_3D ( 'NONE', #17553, #8992, #17456 ) ;
#13600=AXIS2_PLACEMENT_3D ( 'NONE', #16381, #3303, #16108 ) ;
#13619=DIRECTION ( 'NONE',  ( 0.000000000000000000, 0.000000000000000000, 1.000000000000000000 ) ) ;
#13621=EDGE_CURVE ( 'NONE', #17766, #5913, #3491, .T. ) ;
#13625=DIRECTION ( 'NONE',  ( -0.000000000000000000, -1.000000000000000000, -0.000000000000000000 ) ) ;
#13633=AXIS2_PLACEMENT_3D ( 'NONE', #13279, #7713, #864 ) ;
#13636=ORIENTED_EDGE ( 'NONE', *, *, #9701, .F. ) ;
#13641=AXIS2_PLACEMENT_3D ( 'NONE', #7575, #3422, #17000 ) ;
#13643=DIRECTION ( 'NONE',  ( -3.469446951953613696E-16, -0.000000000000000000, -1.000000000000000000 ) ) ;
#13646=FACE_OUTER_BOUND ( 'NONE', #2966, .T. ) ;
#13647=FACE_OUTER_BOUND ( 'NONE', #343, .T. ) ;
#13649=EDGE_LOOP ( 'NONE', ( #567, #14230, #12305, #17334 ) ) ;
#13654=ADVANCED_FACE ( 'NONE', ( #3937 ), #5142, .T. ) ;
#13657=AXIS2_PLACEMENT_3D ( 'NONE', #9314, #13397, #4958 ) ;
#13661=DIRECTION ( 'NONE',  ( 0.000000000000000000, 0.000000000000000000, -1.000000000000000000 ) ) ;
#13668=DIRECTION ( 'NONE',  ( 0.000000000000000000, 0.000000000000000000, 1.000000000000000000 ) ) ;
#13673=ORIENTED_EDGE ( 'NONE', *, *, #8265, .T. ) ;
#13674=CIRCLE ( 'NONE', #14883, 0.9999999999999991118 ) ;
#13676=EDGE_CURVE ( 'NONE', #12007, #15972, #15076, .T. ) ;
#13688=DIRECTION ( 'NONE',  ( -0.000000000000000000, -1.000000000000000000, -0.000000000000000000 ) ) ;
#13690=ORIENTED_EDGE ( 'NONE', *, *, #5542, .F. ) ;
#13691=CARTESIAN_POINT ( 'NONE',  ( -1.734723475976807094E-15, 36.39999999999999147, -2.500000000000000000 ) ) ;
#13694=AXIS2_PLACEMENT_3D ( 'NONE', #7673, #6198, #8881 ) ;
#13697=VERTEX_POINT ( 'NONE', #3331 ) ;
#13700=( LENGTH_UNIT ( ) NAMED_UNIT ( * ) SI_UNIT ( .MILLI., .METRE. ) );
#13708=CIRCLE ( 'NONE', #1881, 0.9999999999999991118 ) ;
#13710=TOROIDAL_SURFACE ( 'NONE', #12815, 9.000000000000001776, 0.9999999999999991118 ) ;
#13715=CARTESIAN_POINT ( 'NONE',  ( -1.734723475976807094E-15, 20.99999999999999289, -11.50000000000000178 ) ) ;
#13719=AXIS2_PLACEMENT_3D ( 'NONE', #14818, #3406, #10438 ) ;
#13720=( NAMED_UNIT ( * ) PLANE_ANGLE_UNIT ( ) SI_UNIT ( $, .RADIAN. ) );
#13730=ORIENTED_EDGE ( 'NONE', *, *, #8407, .F. ) ;
#13737=LINE ( 'NONE', #77, #11447 ) ;
#13738=CARTESIAN_POINT ( 'NONE',  ( -1.734723475976807094E-15, 34.19999999999999574, -11.50000000000000178 ) ) ;
#13739=FACE_OUTER_BOUND ( 'NONE', #15537, .T. ) ;
#13741=VERTEX_POINT ( 'NONE', #18057 ) ;
#13742=DIRECTION ( 'NONE',  ( 1.000000000000000000, 0.000000000000000000, -4.336808689942021680E-16 ) ) ;
#13744=EDGE_CURVE ( 'NONE', #904, #12007, #17119, .T. ) ;
#13747=EDGE_LOOP ( 'NONE', ( #16942, #14541, #11734, #10223 ) ) ;
#13749=EDGE_CURVE ( 'NONE', #17274, #11085, #13847, .T. ) ;
#13754=DIRECTION ( 'NONE',  ( 1.000000000000000000, 0.000000000000000000, -4.336808689942021680E-16 ) ) ;
#13755=DIRECTION ( 'NONE',  ( -3.469446951953613696E-16, -0.000000000000000000, -1.000000000000000000 ) ) ;
#13759=DIRECTION ( 'NONE',  ( 0.000000000000000000, 0.000000000000000000, -1.000000000000000000 ) ) ;
#13767=DIRECTION ( 'NONE',  ( 0.000000000000000000, 0.000000000000000000, -1.000000000000000000 ) ) ;
#13774=ORIENTED_EDGE ( 'NONE', *, *, #16926, .F. ) ;
#13775=MANIFOLD_SOLID_BREP ( 'LPattern6[8]', #9404 ) ;
#13783=CARTESIAN_POINT ( 'NONE',  ( 9.000000000000005329, 16.59999999999999787, 2.499999999999997335 ) ) ;
#13787=ORIENTED_EDGE ( 'NONE', *, *, #870, .T. ) ;
#13794=CIRCLE ( 'NONE', #15001, 8.000000000000001776 ) ;
#13800=ORIENTED_EDGE ( 'NONE', *, *, #4861, .F. ) ;
#13802=DIRECTION ( 'NONE',  ( 0.000000000000000000, 0.000000000000000000, -1.000000000000000000 ) ) ;
#13807=MANIFOLD_SOLID_BREP ( 'LPattern6[3]', #10585 ) ;
#13808=DIRECTION ( 'NONE',  ( -3.469446951953613696E-16, -0.000000000000000000, -1.000000000000000000 ) ) ;
#13814=ORIENTED_EDGE ( 'NONE', *, *, #2798, .T. ) ;
#13823=EDGE_LOOP ( 'NONE', ( #132, #1592, #15054, #16688 ) ) ;
#13827=( LENGTH_UNIT ( ) NAMED_UNIT ( * ) SI_UNIT ( .MILLI., .METRE. ) );
#13830=CARTESIAN_POINT ( 'NONE',  ( -1.734723475976807094E-15, 36.39999999999999147, -10.50000000000000178 ) ) ;
#13834=CARTESIAN_POINT ( 'NONE',  ( -9.000000000000001776, 31.99999999999999289, 2.499999999999995559 ) ) ;
#13845=CLOSED_SHELL ( 'NONE', ( #5724, #4390, #10064, #15065, #12553, #9652, #8267, #13503, #1874, #8459 ) ) ;
#13846=EDGE_CURVE ( 'NONE', #5635, #6645, #2907, .T. ) ;
#13847=CIRCLE ( 'NONE', #15043, 0.9999999999999991118 ) ;
#13848=ADVANCED_FACE ( 'NONE', ( #1526 ), #16087, .T. ) ;
#13849=CIRCLE ( 'NONE', #14451, 0.9999999999999991118 ) ;
#13853=CARTESIAN_POINT ( 'NONE',  ( -9.000000000000001776, 18.79999999999999361, 2.499999999999998224 ) ) ;
#13857=CARTESIAN_POINT ( 'NONE',  ( -8.000000000000001776, 43.00000000000000000, 2.499999999999995115 ) ) ;
#13863=TOROIDAL_SURFACE ( 'NONE', #16247, 9.000000000000001776, 0.9999999999999991118 ) ;
#13865=TOROIDAL_SURFACE ( 'NONE', #8234, 9.000000000000003553, 0.9999999999999991118 ) ;
#13874=DIRECTION ( 'NONE',  ( -1.000000000000000000, 0.000000000000000000, 4.336808689942021680E-16 ) ) ;
#13875=AXIS2_PLACEMENT_3D ( 'NONE', #15032, #14763, #16515 ) ;
#13876=CARTESIAN_POINT ( 'NONE',  ( -1.734723475976807094E-15, 43.00000000000000000, -2.500000000000000000 ) ) ;
#13887=DIRECTION ( 'NONE',  ( 0.000000000000000000, 0.000000000000000000, 1.000000000000000000 ) ) ;
#13897=DIRECTION ( 'NONE',  ( 1.000000000000000000, 0.000000000000000000, 0.000000000000000000 ) ) ;
#13900=ORIENTED_EDGE ( 'NONE', *, *, #9442, .T. ) ;
#13905=EDGE_LOOP ( 'NONE', ( #3733, #8172, #6569, #4455 ) ) ;
#13909=ORIENTED_EDGE ( 'NONE', *, *, #9977, .F. ) ;
#13926=( NAMED_UNIT ( * ) PLANE_ANGLE_UNIT ( ) SI_UNIT ( $, .RADIAN. ) );
#13927=CARTESIAN_POINT ( 'NONE',  ( 9.000000000000001776, 20.99999999999999289, -2.500000000000002665 ) ) ;
#13932=DIRECTION ( 'NONE',  ( 0.000000000000000000, 0.000000000000000000, -1.000000000000000000 ) ) ;
#13934=CIRCLE ( 'NONE', #3855, 0.9999999999999991118 ) ;
#13940=DIRECTION ( 'NONE',  ( -1.000000000000000000, 0.000000000000000000, 4.336808689942021680E-16 ) ) ;
#13949=CYLINDRICAL_SURFACE ( 'NONE', #18046, 0.9999999999999991118 ) ;
#13952=ADVANCED_FACE ( 'NONE', ( #17589 ), #13863, .T. ) ;
#13958=DIRECTION ( 'NONE',  ( -3.469446951953613696E-16, -0.000000000000000000, -1.000000000000000000 ) ) ;
#13961=CARTESIAN_POINT ( 'NONE',  ( -9.000000000000001776, 20.99999999999999289, 2.499999999999998224 ) ) ;
#13976=EDGE_CURVE ( 'NONE', #10092, #5374, #6459, .T. ) ;
#13991=ORIENTED_EDGE ( 'NONE', *, *, #14255, .F. ) ;
#14004=ORIENTED_EDGE ( 'NONE', *, *, #4226, .T. ) ;
#14012=MECHANICAL_DESIGN_GEOMETRIC_PRESENTATION_REPRESENTATION('',(#6355),#3087);
#14019=FACE_OUTER_BOUND ( 'NONE', #3871, .T. ) ;
#14020=DIRECTION ( 'NONE',  ( 0.000000000000000000, 0.000000000000000000, -1.000000000000000000 ) ) ;
#14030=AXIS2_PLACEMENT_3D ( 'NONE', #2371, #15340, #13754 ) ;
#14033=DIRECTION ( 'NONE',  ( -3.469446951953613696E-16, -0.000000000000000000, -1.000000000000000000 ) ) ;
#14044=ORIENTED_EDGE ( 'NONE', *, *, #314, .F. ) ;
#14058=FACE_OUTER_BOUND ( 'NONE', #9567, .T. ) ;
#14066=( NAMED_UNIT ( * ) PLANE_ANGLE_UNIT ( ) SI_UNIT ( $, .RADIAN. ) );
#14067=FACE_OUTER_BOUND ( 'NONE', #15684, .T. ) ;
#14069=EDGE_CURVE ( 'NONE', #5475, #4719, #9207, .T. ) ;
#14071=DIRECTION ( 'NONE',  ( -0.000000000000000000, -1.000000000000000000, -0.000000000000000000 ) ) ;
#14076=DIRECTION ( 'NONE',  ( 0.000000000000000000, 0.000000000000000000, 1.000000000000000000 ) ) ;
#14077=ORIENTED_EDGE ( 'NONE', *, *, #3605, .T. ) ;
#14079=VECTOR ( 'NONE', #4746, 1000.000000000000000 ) ;
#14092=EDGE_CURVE ( 'NONE', #15689, #13741, #694, .T. ) ;
#14095=CIRCLE ( 'NONE', #14392, 0.9999999999999991118 ) ;
#14105=ORIENTED_EDGE ( 'NONE', *, *, #10176, .F. ) ;
#14107=DIRECTION ( 'NONE',  ( 1.000000000000000000, 0.000000000000000000, -4.336808689942021680E-16 ) ) ;
#14108=DIRECTION ( 'NONE',  ( -0.000000000000000000, -1.000000000000000000, -0.000000000000000000 ) ) ;
#14111=ORIENTED_EDGE ( 'NONE', *, *, #17675, .T. ) ;
#14117=AXIS2_PLACEMENT_3D ( 'NONE', #882, #14804, #7731 ) ;
#14118=CARTESIAN_POINT ( 'NONE',  ( -1.734723475976807094E-15, 16.59999999999999787, -2.500000000000000000 ) ) ;
#14120=DIRECTION ( 'NONE',  ( 0.000000000000000000, 0.000000000000000000, -1.000000000000000000 ) ) ;
#14127=ORIENTED_EDGE ( 'NONE', *, *, #15232, .T. ) ;
#14140=DIRECTION ( 'NONE',  ( -4.915049848600951133E-16, 0.000000000000000000, -1.000000000000000000 ) ) ;
#14153=DIRECTION ( 'NONE',  ( -1.000000000000000000, 0.000000000000000000, 4.336808689942021680E-16 ) ) ;
#14155=DIRECTION ( 'NONE',  ( -0.000000000000000000, -1.000000000000000000, -0.000000000000000000 ) ) ;
#14160=AXIS2_PLACEMENT_3D ( 'NONE', #4574, #4388, #5694 ) ;
#14167=DIRECTION ( 'NONE',  ( 1.000000000000000000, 0.000000000000000000, 0.000000000000000000 ) ) ;
#14172=ORIENTED_EDGE ( 'NONE', *, *, #11576, .F. ) ;
#14176=AXIS2_PLACEMENT_3D ( 'NONE', #7567, #10629, #3589 ) ;
#14191=CIRCLE ( 'NONE', #3830, 0.9999999999999991118 ) ;
#14195=DIRECTION ( 'NONE',  ( 3.469446951953612217E-16, -0.000000000000000000, 1.000000000000000000 ) ) ;
#14196=ORIENTED_EDGE ( 'NONE', *, *, #2416, .F. ) ;
#14197=VERTEX_POINT ( 'NONE', #8176 ) ;
#14208=VECTOR ( 'NONE', #6064, 1000.000000000000000 ) ;
#14214=MANIFOLD_SOLID_BREP ( 'LPattern6[10]', #13845 ) ;
#14217=CIRCLE ( 'NONE', #13031, 10.00000000000000000 ) ;
#14222=DIRECTION ( 'NONE',  ( 0.000000000000000000, 0.000000000000000000, -1.000000000000000000 ) ) ;
#14223=ORIENTED_EDGE ( 'NONE', *, *, #8513, .T. ) ;
#14224=ADVANCED_FACE ( 'NONE', ( #17091 ), #12080, .T. ) ;
#14226=FACE_OUTER_BOUND ( 'NONE', #4177, .T. ) ;
#14229=DIRECTION ( 'NONE',  ( 0.000000000000000000, 0.000000000000000000, -1.000000000000000000 ) ) ;
#14230=ORIENTED_EDGE ( 'NONE', *, *, #18063, .T. ) ;
#14232=CIRCLE ( 'NONE', #7703, 0.9999999999999991118 ) ;
#14237=CARTESIAN_POINT ( 'NONE',  ( 0.000000000000000000, 23.19999999999999574, 2.500000000000000000 ) ) ;
#14239=CARTESIAN_POINT ( 'NONE',  ( -1.734723475976807094E-15, 18.79999999999999361, -2.500000000000000000 ) ) ;
#14245=ORIENTED_EDGE ( 'NONE', *, *, #12728, .T. ) ;
#14255=EDGE_CURVE ( 'NONE', #10347, #17611, #16847, .T. ) ;
#14265=FACE_OUTER_BOUND ( 'NONE', #2134, .T. ) ;
#14275=VERTEX_POINT ( 'NONE', #14679 ) ;
#14279=AXIS2_PLACEMENT_3D ( 'NONE', #4318, #13029, #14153 ) ;
#14283=DIRECTION ( 'NONE',  ( -1.000000000000000000, 0.000000000000000000, 4.336808689942021680E-16 ) ) ;
#14292=DIRECTION ( 'NONE',  ( -3.469446951953613696E-16, -0.000000000000000000, -1.000000000000000000 ) ) ;
#14306=VECTOR ( 'NONE', #2410, 1000.000000000000000 ) ;
#14307=TOROIDAL_SURFACE ( 'NONE', #9277, 9.000000000000001776, 0.9999999999999991118 ) ;
#14314=DIRECTION ( 'NONE',  ( 3.469446951953612217E-16, -0.000000000000000000, 1.000000000000000000 ) ) ;
#14316=EDGE_CURVE ( 'NONE', #14997, #14652, #3227, .T. ) ;
#14321=VECTOR ( 'NONE', #16388, 1000.000000000000000 ) ;
#14332=DIRECTION ( 'NONE',  ( 0.000000000000000000, 0.000000000000000000, 1.000000000000000000 ) ) ;
#14347=EDGE_LOOP ( 'NONE', ( #4905, #1760, #18218, #18174 ) ) ;
#14371=CARTESIAN_POINT ( 'NONE',  ( -1.734723475976807094E-15, 34.19999999999999574, -11.50000000000000178 ) ) ;
#14376=CARTESIAN_POINT ( 'NONE',  ( -1.734723475976807094E-15, 16.59999999999999787, -11.50000000000000178 ) ) ;
#14381=DIRECTION ( 'NONE',  ( -1.000000000000000000, 0.000000000000000000, 4.336808689942021680E-16 ) ) ;
#14383=CARTESIAN_POINT ( 'NONE',  ( -1.734723475976807094E-15, 29.79999999999999716, -12.50000000000000000 ) ) ;
#14384=ORIENTED_EDGE ( 'NONE', *, *, #15852, .T. ) ;
#14390=FACE_OUTER_BOUND ( 'NONE', #7775, .T. ) ;
#14392=AXIS2_PLACEMENT_3D ( 'NONE', #3835, #12629, #18045 ) ;
#14394=CIRCLE ( 'NONE', #8449, 8.000000000000003553 ) ;
#14395=CARTESIAN_POINT ( 'NONE',  ( -10.00000000000000000, 18.79999999999999361, 2.499999999999996003 ) ) ;
#14397=DIRECTION ( 'NONE',  ( -1.000000000000000000, 0.000000000000000000, 0.000000000000000000 ) ) ;
#14398=CARTESIAN_POINT ( 'NONE',  ( 8.000000000000005329, 23.19999999999999574, 2.499999999999997780 ) ) ;
#14402=DIRECTION ( 'NONE',  ( 0.000000000000000000, 0.000000000000000000, -1.000000000000000000 ) ) ;
#14403=ORIENTED_EDGE ( 'NONE', *, *, #17630, .T. ) ;
#14405=AXIS2_PLACEMENT_3D ( 'NONE', #15543, #18251, #51 ) ;
#14407=CARTESIAN_POINT ( 'NONE',  ( 9.000000000000000000, 31.99999999999999289, -2.500000000000001332 ) ) ;
#14409=CARTESIAN_POINT ( 'NONE',  ( 9.999999999999998224, 23.19999999999999574, -2.500000000000001776 ) ) ;
#14410=DIRECTION ( 'NONE',  ( 0.000000000000000000, 0.000000000000000000, 1.000000000000000000 ) ) ;
#14412=ORIENTED_EDGE ( 'NONE', *, *, #6327, .T. ) ;
#14417=EDGE_CURVE ( 'NONE', #18202, #15889, #14782, .T. ) ;
#14419=TOROIDAL_SURFACE ( 'NONE', #14729, 9.000000000000001776, 0.9999999999999991118 ) ;
#14423=CARTESIAN_POINT ( 'NONE',  ( -9.000000000000001776, 31.99999999999999289, 2.499999999999998224 ) ) ;
#14432=DIRECTION ( 'NONE',  ( 0.000000000000000000, 0.000000000000000000, -1.000000000000000000 ) ) ;
#14434=CIRCLE ( 'NONE', #1750, 10.00000000000000000 ) ;
#14436=AXIS2_PLACEMENT_3D ( 'NONE', #12839, #8306, #1631 ) ;
#14442=ORIENTED_EDGE ( 'NONE', *, *, #12488, .T. ) ;
#14444=CLOSED_SHELL ( 'NONE', ( #3670, #14669, #9494, #17053, #5804, #9947, #14224, #5195, #18142, #2994 ) ) ;
#14451=AXIS2_PLACEMENT_3D ( 'NONE', #8791, #8603, #377 ) ;
#14453=CARTESIAN_POINT ( 'NONE',  ( 0.000000000000000000, 31.99999999999999289, 2.500000000000000000 ) ) ;
#14456=FACE_OUTER_BOUND ( 'NONE', #16990, .T. ) ;
#14461=LINE ( 'NONE', #1763, #16373 ) ;
#14481=CIRCLE ( 'NONE', #2655, 8.000000000000003553 ) ;
#14483=AXIS2_PLACEMENT_3D ( 'NONE', #8523, #12614, #5663 ) ;
#14488=ORIENTED_EDGE ( 'NONE', *, *, #11743, .T. ) ;
#14493=ADVANCED_FACE ( 'NONE', ( #13646 ), #10683, .T. ) ;
#14497=CIRCLE ( 'NONE', #18058, 0.9999999999999991118 ) ;
#14501=CARTESIAN_POINT ( 'NONE',  ( 8.000000000000001776, 43.00000000000000000, -2.500000000000002220 ) ) ;
#14512=LINE ( 'NONE', #9946, #10712 ) ;
#14526=EDGE_CURVE ( 'NONE', #15102, #12786, #10614, .T. ) ;
#14532=EDGE_CURVE ( 'NONE', #12253, #14997, #12343, .T. ) ;
#14533=CARTESIAN_POINT ( 'NONE',  ( -10.00000000000000000, 27.59999999999999432, 2.499999999999998224 ) ) ;
#14541=ORIENTED_EDGE ( 'NONE', *, *, #17696, .T. ) ;
#14545=CIRCLE ( 'NONE', #8586, 10.00000000000000000 ) ;
#14546=CARTESIAN_POINT ( 'NONE',  ( -1.734723475976807094E-15, 34.19999999999999574, -10.50000000000000178 ) ) ;
#14549=ADVANCED_FACE ( 'NONE', ( #18220 ), #8270, .T. ) ;
#14550=ORIENTED_EDGE ( 'NONE', *, *, #14316, .F. ) ;
#14552=ADVANCED_FACE ( 'NONE', ( #14973 ), #16449, .T. ) ;
#14568=FACE_OUTER_BOUND ( 'NONE', #9362, .T. ) ;
#14573=DIRECTION ( 'NONE',  ( -0.000000000000000000, -1.000000000000000000, -0.000000000000000000 ) ) ;
#14578=DIRECTION ( 'NONE',  ( -3.373073425510457965E-16, 0.000000000000000000, -1.000000000000000000 ) ) ;
#14580=ORIENTED_EDGE ( 'NONE', *, *, #3989, .T. ) ;
#14582=CARTESIAN_POINT ( 'NONE',  ( -9.000000000000001776, 29.79999999999999716, 2.499999999999998224 ) ) ;
#14592=CARTESIAN_POINT ( 'NONE',  ( -1.734723475976807094E-15, 23.19999999999999574, -12.50000000000000000 ) ) ;
#14594=AXIS2_PLACEMENT_3D ( 'NONE', #11444, #15731, #3123 ) ;
#14595=DIRECTION ( 'NONE',  ( 0.000000000000000000, 0.000000000000000000, 1.000000000000000000 ) ) ;
#14597=DIRECTION ( 'NONE',  ( 0.000000000000000000, 0.000000000000000000, -1.000000000000000000 ) ) ;
#14601=EDGE_CURVE ( 'NONE', #4985, #13486, #15964, .T. ) ;
#14602=DIRECTION ( 'NONE',  ( 1.000000000000000000, 0.000000000000000000, -4.336808689942021680E-16 ) ) ;
#14612=TOROIDAL_SURFACE ( 'NONE', #11033, 9.000000000000003553, 0.9999999999999991118 ) ;
#14614=CIRCLE ( 'NONE', #993, 0.9999999999999991118 ) ;
#14620=DIRECTION ( 'NONE',  ( -0.000000000000000000, -1.000000000000000000, -0.000000000000000000 ) ) ;
#14621=MANIFOLD_SOLID_BREP ( 'LPattern6[6]', #16230 ) ;
#14638=ORIENTED_EDGE ( 'NONE', *, *, #4950, .T. ) ;
#14639=AXIS2_PLACEMENT_3D ( 'NONE', #8281, #6522, #17862 ) ;
#14640=CARTESIAN_POINT ( 'NONE',  ( -1.734723475976807094E-15, 38.59999999999999432, -2.500000000000000000 ) ) ;
#14641=DIRECTION ( 'NONE',  ( -0.000000000000000000, -1.000000000000000000, -0.000000000000000000 ) ) ;
#14647=ORIENTED_EDGE ( 'NONE', *, *, #11683, .T. ) ;
#14650=TOROIDAL_SURFACE ( 'NONE', #5748, 9.000000000000001776, 0.9999999999999991118 ) ;
#14652=VERTEX_POINT ( 'NONE', #4155 ) ;
#14655=DIRECTION ( 'NONE',  ( 0.000000000000000000, 0.000000000000000000, 1.000000000000000000 ) ) ;
#14659=MANIFOLD_SOLID_BREP ( 'LPattern6[11]', #14444 ) ;
#14668=CARTESIAN_POINT ( 'NONE',  ( -8.000000000000003553, 25.39999999999999503, -2.500000000000001776 ) ) ;
#14669=ADVANCED_FACE ( 'NONE', ( #14067 ), #5004, .T. ) ;
#14674=ORIENTED_EDGE ( 'NONE', *, *, #15884, .T. ) ;
#14677=DIRECTION ( 'NONE',  ( 0.000000000000000000, 0.000000000000000000, -1.000000000000000000 ) ) ;
#14679=CARTESIAN_POINT ( 'NONE',  ( -10.00000000000000178, 16.59999999999999787, -2.500000000000001776 ) ) ;
#14680=ORIENTED_EDGE ( 'NONE', *, *, #6701, .F. ) ;
#14682=DIRECTION ( 'NONE',  ( 0.000000000000000000, 0.000000000000000000, -1.000000000000000000 ) ) ;
#14690=DIRECTION ( 'NONE',  ( -3.469446951953613696E-16, -0.000000000000000000, -1.000000000000000000 ) ) ;
#14691=LINE ( 'NONE', #16444, #17099 ) ;
#14694=ORIENTED_EDGE ( 'NONE', *, *, #17675, .F. ) ;
#14704=CIRCLE ( 'NONE', #3738, 0.9999999999999991118 ) ;
#14706=AXIS2_PLACEMENT_3D ( 'NONE', #18004, #5274, #6844 ) ;
#14709=CARTESIAN_POINT ( 'NONE',  ( -10.00000000000000000, 36.39999999999999147, 2.499999999999996003 ) ) ;
#14713=CARTESIAN_POINT ( 'NONE',  ( -9.000000000000003553, 36.39999999999999147, -2.500000000000001776 ) ) ;
#14716=CARTESIAN_POINT ( 'NONE',  ( -1.734723475976807094E-15, 34.19999999999999574, -2.500000000000000000 ) ) ;
#14724=CARTESIAN_POINT ( 'NONE',  ( 0.000000000000000000, 34.19999999999999574, 2.500000000000000000 ) ) ;
#14729=AXIS2_PLACEMENT_3D ( 'NONE', #6704, #5683, #14120 ) ;
#14730=EDGE_LOOP ( 'NONE', ( #3691, #6636, #6191, #3960 ) ) ;
#14735=DIRECTION ( 'NONE',  ( -0.000000000000000000, -1.000000000000000000, -0.000000000000000000 ) ) ;
#14739=EDGE_LOOP ( 'NONE', ( #8269, #4153, #9245, #1583 ) ) ;
#14745=ORIENTED_EDGE ( 'NONE', *, *, #8865, .T. ) ;
#14756=CIRCLE ( 'NONE', #7909, 0.9999999999999991118 ) ;
#14758=AXIS2_PLACEMENT_3D ( 'NONE', #7267, #1924, #4498 ) ;
#14760=DIRECTION ( 'NONE',  ( -0.000000000000000000, -1.000000000000000000, -0.000000000000000000 ) ) ;
#14763=DIRECTION ( 'NONE',  ( 0.000000000000000000, 0.000000000000000000, 1.000000000000000000 ) ) ;
#14764=ORIENTED_EDGE ( 'NONE', *, *, #11571, .T. ) ;
#14767=DIRECTION ( 'NONE',  ( 0.000000000000000000, 0.000000000000000000, -1.000000000000000000 ) ) ;
#14773=DIRECTION ( 'NONE',  ( 0.000000000000000000, 0.000000000000000000, -1.000000000000000000 ) ) ;
#14782=CIRCLE ( 'NONE', #2641, 0.9999999999999991118 ) ;
#14785=EDGE_CURVE ( 'NONE', #17369, #7045, #8844, .T. ) ;
#14798=TOROIDAL_SURFACE ( 'NONE', #5299, 9.000000000000003553, 0.9999999999999991118 ) ;
#14804=DIRECTION ( 'NONE',  ( 0.000000000000000000, 0.000000000000000000, 1.000000000000000000 ) ) ;
#14805=CIRCLE ( 'NONE', #4132, 0.9999999999999991118 ) ;
#14807=AXIS2_PLACEMENT_3D ( 'NONE', #1869, #17648, #7499 ) ;
#14808=DIRECTION ( 'NONE',  ( 0.000000000000000000, 0.000000000000000000, -1.000000000000000000 ) ) ;
#14818=CARTESIAN_POINT ( 'NONE',  ( 0.000000000000000000, 38.59999999999999432, 2.500000000000000000 ) ) ;
#14822=CIRCLE ( 'NONE', #6801, 0.9999999999999991118 ) ;
#14825=ORIENTED_EDGE ( 'NONE', *, *, #3723, .F. ) ;
#14829=DIRECTION ( 'NONE',  ( -4.915049848600951133E-16, 0.000000000000000000, -1.000000000000000000 ) ) ;
#14835=EDGE_CURVE ( 'NONE', #11426, #17611, #2653, .T. ) ;
#14849=ORIENTED_EDGE ( 'NONE', *, *, #8513, .F. ) ;
#14852=ORIENTED_EDGE ( 'NONE', *, *, #520, .T. ) ;
#14860=EDGE_CURVE ( 'NONE', #17338, #9655, #9436, .T. ) ;
#14869=ADVANCED_FACE ( 'NONE', ( #4698 ), #14798, .T. ) ;
#14877=DIRECTION ( 'NONE',  ( 0.000000000000000000, 0.000000000000000000, -1.000000000000000000 ) ) ;
#14883=AXIS2_PLACEMENT_3D ( 'NONE', #14407, #1713, #12911 ) ;
#14899=EDGE_CURVE ( 'NONE', #1204, #7975, #18360, .T. ) ;
#14900=DIRECTION ( 'NONE',  ( 0.000000000000000000, 0.000000000000000000, -1.000000000000000000 ) ) ;
#14901=EDGE_CURVE ( 'NONE', #8582, #16215, #14497, .T. ) ;
#14903=CARTESIAN_POINT ( 'NONE',  ( 0.000000000000000000, 25.39999999999999503, 2.500000000000000000 ) ) ;
#14912=CARTESIAN_POINT ( 'NONE',  ( -1.734723475976807094E-15, 31.99999999999999289, -12.50000000000000000 ) ) ;
#14919=ORIENTED_EDGE ( 'NONE', *, *, #10738, .F. ) ;
#14922=ORIENTED_EDGE ( 'NONE', *, *, #4423, .T. ) ;
#14923=CARTESIAN_POINT ( 'NONE',  ( -1.734723475976807094E-15, 23.19999999999999574, -2.500000000000000000 ) ) ;
#14931=ORIENTED_EDGE ( 'NONE', *, *, #10461, .T. ) ;
#14934=ORIENTED_EDGE ( 'NONE', *, *, #7209, .F. ) ;
#14941=AXIS2_PLACEMENT_3D ( 'NONE', #7723, #6347, #17683 ) ;
#14942=VERTEX_POINT ( 'NONE', #9149 ) ;
#14945=ORIENTED_EDGE ( 'NONE', *, *, #18083, .F. ) ;
#14946=DIRECTION ( 'NONE',  ( -0.000000000000000000, -1.000000000000000000, -0.000000000000000000 ) ) ;
#14953=ORIENTED_EDGE ( 'NONE', *, *, #6552, .T. ) ;
#14957=ORIENTED_EDGE ( 'NONE', *, *, #10461, .F. ) ;
#14959=CARTESIAN_POINT ( 'NONE',  ( 0.000000000000000000, 27.59999999999999432, 2.500000000000000000 ) ) ;
#14970=CARTESIAN_POINT ( 'NONE',  ( -1.734723475976807094E-15, 31.99999999999999289, -10.50000000000000178 ) ) ;
#14973=FACE_OUTER_BOUND ( 'NONE', #2237, .T. ) ;
#14988=CARTESIAN_POINT ( 'NONE',  ( -8.000000000000003553, 16.59999999999999787, -2.500000000000001776 ) ) ;
#14990=ORIENTED_EDGE ( 'NONE', *, *, #18293, .F. ) ;
#14993=EDGE_CURVE ( 'NONE', #10845, #1108, #5882, .T. ) ;
#14997=VERTEX_POINT ( 'NONE', #3501 ) ;
#15000=ORIENTED_EDGE ( 'NONE', *, *, #11021, .T. ) ;
#15001=AXIS2_PLACEMENT_3D ( 'NONE', #14118, #1430, #15790 ) ;
#15011=FACE_OUTER_BOUND ( 'NONE', #5460, .T. ) ;
#15014=ORIENTED_EDGE ( 'NONE', *, *, #17032, .T. ) ;
#15020=CIRCLE ( 'NONE', #4326, 8.000000000000003553 ) ;
#15031=ADVANCED_FACE ( 'NONE', ( #9415 ), #877, .T. ) ;
#15032=CARTESIAN_POINT ( 'NONE',  ( -9.000000000000003553, 43.00000000000000000, -2.500000000000001776 ) ) ;
#15043=AXIS2_PLACEMENT_3D ( 'NONE', #5776, #15446, #10028 ) ;
#15049=AXIS2_PLACEMENT_3D ( 'NONE', #11155, #9771, #12277 ) ;
#15053=CYLINDRICAL_SURFACE ( 'NONE', #7937, 0.9999999999999991118 ) ;
#15054=ORIENTED_EDGE ( 'NONE', *, *, #18293, .T. ) ;
#15065=ADVANCED_FACE ( 'NONE', ( #2124 ), #10812, .T. ) ;
#15066=DIRECTION ( 'NONE',  ( 0.000000000000000000, 0.000000000000000000, 1.000000000000000000 ) ) ;
#15070=CARTESIAN_POINT ( 'NONE',  ( 0.000000000000000000, 16.59999999999999787, 2.500000000000000000 ) ) ;
#15073=CARTESIAN_POINT ( 'NONE',  ( 8.000000000000000000, 23.19999999999999574, -2.500000000000000888 ) ) ;
#15076=LINE ( 'NONE', #13857, #4654 ) ;
#15080=DIRECTION ( 'NONE',  ( -0.000000000000000000, -1.000000000000000000, -0.000000000000000000 ) ) ;
#15091=DIRECTION ( 'NONE',  ( -1.000000000000000000, 0.000000000000000000, 4.336808689942021680E-16 ) ) ;
#15094=DIRECTION ( 'NONE',  ( 0.000000000000000000, 0.000000000000000000, 1.000000000000000000 ) ) ;
#15102=VERTEX_POINT ( 'NONE', #10445 ) ;
#15103=EDGE_LOOP ( 'NONE', ( #2807, #1802, #16952, #6016 ) ) ;
#15107=CARTESIAN_POINT ( 'NONE',  ( 10.00000000000000000, 25.39999999999999503, -2.500000000000003109 ) ) ;
#15109=ORIENTED_EDGE ( 'NONE', *, *, #9303, .T. ) ;
#15112=ORIENTED_EDGE ( 'NONE', *, *, #10152, .F. ) ;
#15119=CIRCLE ( 'NONE', #12732, 0.9999999999999991118 ) ;
#15123=DIRECTION ( 'NONE',  ( -0.000000000000000000, -1.000000000000000000, -0.000000000000000000 ) ) ;
#15128=ORIENTED_EDGE ( 'NONE', *, *, #13288, .F. ) ;
#15133=AXIS2_PLACEMENT_3D ( 'NONE', #4002, #2536, #9469 ) ;
#15141=VECTOR ( 'NONE', #13206, 1000.000000000000000 ) ;
#15147=DIRECTION ( 'NONE',  ( 3.469446951953612217E-16, -0.000000000000000000, 1.000000000000000000 ) ) ;
#15148=DIRECTION ( 'NONE',  ( 0.000000000000000000, 0.000000000000000000, -1.000000000000000000 ) ) ;
#15156=CARTESIAN_POINT ( 'NONE',  ( -1.734723475976807094E-15, 20.99999999999999289, -10.50000000000000178 ) ) ;
#15157=FACE_OUTER_BOUND ( 'NONE', #5347, .T. ) ;
#15161=ADVANCED_FACE ( 'NONE', ( #16672 ), #15663, .T. ) ;
#15166=VERTEX_POINT ( 'NONE', #2756 ) ;
#15172=CARTESIAN_POINT ( 'NONE',  ( -8.000000000000001776, 36.39999999999999147, 2.499999999999998224 ) ) ;
#15187=DIRECTION ( 'NONE',  ( 0.000000000000000000, 0.000000000000000000, 1.000000000000000000 ) ) ;
#15189=FACE_OUTER_BOUND ( 'NONE', #1147, .T. ) ;
#15191=ORIENTED_EDGE ( 'NONE', *, *, #137, .F. ) ;
#15193=CIRCLE ( 'NONE', #4821, 0.9999999999999991118 ) ;
#15197=EDGE_LOOP ( 'NONE', ( #8801, #9043, #7017, #7344 ) ) ;
#15209=ORIENTED_EDGE ( 'NONE', *, *, #10220, .F. ) ;
#15210=CIRCLE ( 'NONE', #7776, 0.9999999999999991118 ) ;
#15216=FACE_OUTER_BOUND ( 'NONE', #15467, .T. ) ;
#15217=ORIENTED_EDGE ( 'NONE', *, *, #3829, .F. ) ;
#15220=TOROIDAL_SURFACE ( 'NONE', #12826, 9.000000000000003553, 0.9999999999999991118 ) ;
#15222=ORIENTED_EDGE ( 'NONE', *, *, #6778, .T. ) ;
#15229=EDGE_CURVE ( 'NONE', #156, #18266, #11801, .T. ) ;
#15232=EDGE_CURVE ( 'NONE', #10052, #13486, #7966, .T. ) ;
#15238=EDGE_CURVE ( 'NONE', #7134, #3136, #2062, .T. ) ;
#15242=DIRECTION ( 'NONE',  ( 0.000000000000000000, 0.000000000000000000, -1.000000000000000000 ) ) ;
#15243=EDGE_LOOP ( 'NONE', ( #13256, #776, #13141, #8922 ) ) ;
#15246=EDGE_CURVE ( 'NONE', #5374, #11211, #12401, .T. ) ;
#15250=ORIENTED_EDGE ( 'NONE', *, *, #15559, .F. ) ;
#15257=FACE_OUTER_BOUND ( 'NONE', #5117, .T. ) ;
#15264=AXIS2_PLACEMENT_3D ( 'NONE', #7453, #10513, #6598 ) ;
#15268=CARTESIAN_POINT ( 'NONE',  ( -1.734723475976807094E-15, 31.99999999999999289, -2.500000000000000000 ) ) ;
#15270=DIRECTION ( 'NONE',  ( -0.000000000000000000, -1.000000000000000000, -0.000000000000000000 ) ) ;
#15272=ORIENTED_EDGE ( 'NONE', *, *, #7679, .F. ) ;
#15276=AXIS2_PLACEMENT_3D ( 'NONE', #4369, #17015, #15436 ) ;
#15281=ORIENTED_EDGE ( 'NONE', *, *, #375, .T. ) ;
#15290=CARTESIAN_POINT ( 'NONE',  ( 9.000000000000000000, 38.59999999999999432, -2.500000000000001332 ) ) ;
#15304=CARTESIAN_POINT ( 'NONE',  ( 8.000000000000001776, 38.59999999999999432, -2.500000000000002220 ) ) ;
#15306=AXIS2_PLACEMENT_3D ( 'NONE', #7934, #12200, #10905 ) ;
#15309=DIRECTION ( 'NONE',  ( 0.000000000000000000, 0.000000000000000000, -1.000000000000000000 ) ) ;
#15310=CARTESIAN_POINT ( 'NONE',  ( -1.734723475976807094E-15, 43.00000000000000000, -10.50000000000000178 ) ) ;
#15311=ORIENTED_EDGE ( 'NONE', *, *, #16427, .T. ) ;
#15320=CIRCLE ( 'NONE', #7594, 10.00000000000000000 ) ;
#15330=DIRECTION ( 'NONE',  ( -0.000000000000000000, -1.000000000000000000, -0.000000000000000000 ) ) ;
#15331=CARTESIAN_POINT ( 'NONE',  ( 9.000000000000001776, 23.19999999999999574, -2.500000000000002665 ) ) ;
#15332=CARTESIAN_POINT ( 'NONE',  ( -10.00000000000000178, 38.59999999999999432, -2.500000000000001776 ) ) ;
#15340=DIRECTION ( 'NONE',  ( 3.469446951953612217E-16, -0.000000000000000000, 1.000000000000000000 ) ) ;
#15341=DIRECTION ( 'NONE',  ( -1.000000000000000000, 0.000000000000000000, 4.336808689942021680E-16 ) ) ;
#15343=CLOSED_SHELL ( 'NONE', ( #14869, #7732, #9879, #3759, #9665, #13049, #2262, #13848, #5112, #10282 ) ) ;
#15346=CYLINDRICAL_SURFACE ( 'NONE', #1407, 0.9999999999999991118 ) ;
#15347=EDGE_CURVE ( 'NONE', #456, #14275, #14805, .T. ) ;
#15349=DIRECTION ( 'NONE',  ( -1.000000000000000000, 0.000000000000000000, 4.336808689942021680E-16 ) ) ;
#15357=DIRECTION ( 'NONE',  ( -3.373073425510457965E-16, 0.000000000000000000, -1.000000000000000000 ) ) ;
#15367=FACE_OUTER_BOUND ( 'NONE', #8152, .T. ) ;
#15370=AXIS2_PLACEMENT_3D ( 'NONE', #9472, #15330, #6689 ) ;
#15372=AXIS2_PLACEMENT_3D ( 'NONE', #15865, #188, #5837 ) ;
#15378=ORIENTED_EDGE ( 'NONE', *, *, #31, .T. ) ;
#15392=EDGE_CURVE ( 'NONE', #723, #3667, #15680, .T. ) ;
#15396=VECTOR ( 'NONE', #13572, 1000.000000000000000 ) ;
#15399=ORIENTED_EDGE ( 'NONE', *, *, #14899, .F. ) ;
#15400=AXIS2_PLACEMENT_3D ( 'NONE', #15544, #8210, #13874 ) ;
#15415=ORIENTED_EDGE ( 'NONE', *, *, #3090, .T. ) ;
#15424=EDGE_CURVE ( 'NONE', #5921, #2131, #8549, .T. ) ;
#15429=CARTESIAN_POINT ( 'NONE',  ( 0.000000000000000000, 23.19999999999999574, 2.500000000000000000 ) ) ;
#15430=ORIENTED_EDGE ( 'NONE', *, *, #16232, .F. ) ;
#15436=DIRECTION ( 'NONE',  ( 0.000000000000000000, 0.000000000000000000, -1.000000000000000000 ) ) ;
#15437=CYLINDRICAL_SURFACE ( 'NONE', #12304, 0.9999999999999991118 ) ;
#15440=CIRCLE ( 'NONE', #2987, 0.9999999999999991118 ) ;
#15441=CARTESIAN_POINT ( 'NONE',  ( -9.000000000000001776, 38.59999999999999432, 2.499999999999995559 ) ) ;
#15442=DIRECTION ( 'NONE',  ( 0.000000000000000000, 0.000000000000000000, 1.000000000000000000 ) ) ;
#15446=DIRECTION ( 'NONE',  ( -1.000000000000000000, 0.000000000000000000, 0.000000000000000000 ) ) ;
#15451=VECTOR ( 'NONE', #10203, 1000.000000000000000 ) ;
#15457=EDGE_CURVE ( 'NONE', #3719, #17766, #2946, .T. ) ;
#15459=DIRECTION ( 'NONE',  ( -0.000000000000000000, -1.000000000000000000, -0.000000000000000000 ) ) ;
#15464=TOROIDAL_SURFACE ( 'NONE', #4485, 9.000000000000001776, 0.9999999999999991118 ) ;
#15467=EDGE_LOOP ( 'NONE', ( #6003, #6262, #746, #9203 ) ) ;
#15475=CIRCLE ( 'NONE', #969, 0.9999999999999991118 ) ;
#15498=AXIS2_PLACEMENT_3D ( 'NONE', #8905, #1887, #14682 ) ;
#15500=AXIS2_PLACEMENT_3D ( 'NONE', #9002, #11964, #14677 ) ;
#15504=CARTESIAN_POINT ( 'NONE',  ( -10.00000000000000178, 43.00000000000000000, -2.500000000000001776 ) ) ;
#15509=CARTESIAN_POINT ( 'NONE',  ( -1.734723475976807094E-15, 34.19999999999999574, -2.500000000000000000 ) ) ;
#15511=EDGE_LOOP ( 'NONE', ( #2852, #13909, #13421, #11557 ) ) ;
#15514=DIRECTION ( 'NONE',  ( -3.469446951953613696E-16, -0.000000000000000000, -1.000000000000000000 ) ) ;
#15525=EDGE_CURVE ( 'NONE', #7134, #17274, #286, .T. ) ;
#15527=DIRECTION ( 'NONE',  ( -1.000000000000000000, 0.000000000000000000, 4.336808689942021680E-16 ) ) ;
#15530=DIRECTION ( 'NONE',  ( -1.000000000000000000, 0.000000000000000000, 4.336808689942021680E-16 ) ) ;
#15536=CARTESIAN_POINT ( 'NONE',  ( -8.000000000000001776, 23.19999999999999574, 2.499999999999995115 ) ) ;
#15537=EDGE_LOOP ( 'NONE', ( #6148, #7989, #8428, #3794 ) ) ;
#15543=CARTESIAN_POINT ( 'NONE',  ( 9.000000000000001776, 38.59999999999999432, -2.500000000000002665 ) ) ;
#15544=CARTESIAN_POINT ( 'NONE',  ( -9.000000000000001776, 23.19999999999999574, 2.499999999999995559 ) ) ;
#15548=ORIENTED_EDGE ( 'NONE', *, *, #5873, .F. ) ;
#15557=ORIENTED_EDGE ( 'NONE', *, *, #6159, .F. ) ;
#15559=EDGE_CURVE ( 'NONE', #1143, #6012, #17479, .T. ) ;
#15561=EDGE_LOOP ( 'NONE', ( #17142, #13346, #11308, #6269 ) ) ;
#15576=AXIS2_PLACEMENT_3D ( 'NONE', #10318, #14410, #15999 ) ;
#15589=DIRECTION ( 'NONE',  ( 3.469446951953612217E-16, -0.000000000000000000, 1.000000000000000000 ) ) ;
#15593=CARTESIAN_POINT ( 'NONE',  ( -1.734723475976807094E-15, 23.19999999999999574, -2.500000000000000000 ) ) ;
#15602=CIRCLE ( 'NONE', #4048, 10.00000000000000000 ) ;
#15603=DIRECTION ( 'NONE',  ( -1.000000000000000000, 0.000000000000000000, 4.336808689942021680E-16 ) ) ;
#15612=CARTESIAN_POINT ( 'NONE',  ( -1.734723475976807094E-15, 16.59999999999999787, -2.500000000000000000 ) ) ;
#15627=CARTESIAN_POINT ( 'NONE',  ( 9.000000000000001776, 43.00000000000000000, -2.500000000000002665 ) ) ;
#15630=CARTESIAN_POINT ( 'NONE',  ( -1.734723475976807094E-15, 27.59999999999999432, -2.500000000000000000 ) ) ;
#15636=AXIS2_PLACEMENT_3D ( 'NONE', #9570, #10595, #17855 ) ;
#15638=AXIS2_PLACEMENT_3D ( 'NONE', #9290, #17937, #4848 ) ;
#15639=ORIENTED_EDGE ( 'NONE', *, *, #3400, .F. ) ;
#15642=CARTESIAN_POINT ( 'NONE',  ( 10.00000000000000355, 16.59999999999999787, 2.499999999999996891 ) ) ;
#15647=VERTEX_POINT ( 'NONE', #14546 ) ;
#15648=( LENGTH_UNIT ( ) NAMED_UNIT ( * ) SI_UNIT ( .MILLI., .METRE. ) );
#15649=CIRCLE ( 'NONE', #12976, 0.9999999999999991118 ) ;
#15650=CARTESIAN_POINT ( 'NONE',  ( -9.000000000000001776, 23.19999999999999574, 2.499999999999998224 ) ) ;
#15657=CARTESIAN_POINT ( 'NONE',  ( -1.734723475976807094E-15, 25.39999999999999503, -2.500000000000000000 ) ) ;
#15663=TOROIDAL_SURFACE ( 'NONE', #7069, 9.000000000000003553, 0.9999999999999991118 ) ;
#15673=AXIS2_PLACEMENT_3D ( 'NONE', #18340, #4133, #48 ) ;
#15678=CYLINDRICAL_SURFACE ( 'NONE', #2222, 0.9999999999999991118 ) ;
#15680=CIRCLE ( 'NONE', #12121, 0.9999999999999991118 ) ;
#15684=EDGE_LOOP ( 'NONE', ( #10146, #8134, #1757, #11488 ) ) ;
#15687=DIRECTION ( 'NONE',  ( -0.000000000000000000, -1.000000000000000000, -0.000000000000000000 ) ) ;
#15688=DIRECTION ( 'NONE',  ( 0.000000000000000000, 0.000000000000000000, -1.000000000000000000 ) ) ;
#15689=VERTEX_POINT ( 'NONE', #3505 ) ;
#15693=AXIS2_PLACEMENT_3D ( 'NONE', #8007, #16840, #15349 ) ;
#15709=DIRECTION ( 'NONE',  ( 1.000000000000000000, 0.000000000000000000, 0.000000000000000000 ) ) ;
#15710=CARTESIAN_POINT ( 'NONE',  ( 8.000000000000000000, 27.59999999999999432, -2.500000000000000888 ) ) ;
#15714=AXIS2_PLACEMENT_3D ( 'NONE', #1365, #56, #2845 ) ;
#15717=EDGE_CURVE ( 'NONE', #9679, #7045, #10449, .T. ) ;
#15718=CYLINDRICAL_SURFACE ( 'NONE', #16348, 0.9999999999999991118 ) ;
#15725=CARTESIAN_POINT ( 'NONE',  ( -9.000000000000003553, 29.79999999999999716, -2.500000000000001776 ) ) ;
#15731=DIRECTION ( 'NONE',  ( -0.000000000000000000, -1.000000000000000000, -0.000000000000000000 ) ) ;
#15736=ORIENTED_EDGE ( 'NONE', *, *, #18236, .F. ) ;
#15739=ORIENTED_EDGE ( 'NONE', *, *, #9598, .F. ) ;
#15742=EDGE_CURVE ( 'NONE', #17338, #4165, #1470, .T. ) ;
#15746=DIRECTION ( 'NONE',  ( 3.469446951953612217E-16, -0.000000000000000000, 1.000000000000000000 ) ) ;
#15775=EDGE_CURVE ( 'NONE', #10347, #12347, #7080, .T. ) ;
#15776=DIRECTION ( 'NONE',  ( -0.000000000000000000, -1.000000000000000000, -0.000000000000000000 ) ) ;
#15783=CARTESIAN_POINT ( 'NONE',  ( -1.734723475976807094E-15, 20.99999999999999289, -11.50000000000000178 ) ) ;
#15790=DIRECTION ( 'NONE',  ( 0.000000000000000000, 0.000000000000000000, -1.000000000000000000 ) ) ;
#15791=ADVANCED_FACE ( 'NONE', ( #18344 ), #4037, .T. ) ;
#15794=CIRCLE ( 'NONE', #4534, 0.9999999999999991118 ) ;
#15796=EDGE_CURVE ( 'NONE', #6366, #9679, #16885, .T. ) ;
#15797=DIRECTION ( 'NONE',  ( 0.000000000000000000, 0.000000000000000000, -1.000000000000000000 ) ) ;
#15799=DIRECTION ( 'NONE',  ( 3.469446951953612217E-16, -0.000000000000000000, 1.000000000000000000 ) ) ;
#15802=ORIENTED_EDGE ( 'NONE', *, *, #11179, .F. ) ;
#15805=DIRECTION ( 'NONE',  ( 3.469446951953612217E-16, -0.000000000000000000, 1.000000000000000000 ) ) ;
#15806=AXIS2_PLACEMENT_3D ( 'NONE', #11252, #4126, #1352 ) ;
#15820=DIRECTION ( 'NONE',  ( -3.469446951953613696E-16, -0.000000000000000000, -1.000000000000000000 ) ) ;
#15835=( LENGTH_UNIT ( ) NAMED_UNIT ( * ) SI_UNIT ( .MILLI., .METRE. ) );
#15838=CARTESIAN_POINT ( 'NONE',  ( 10.00000000000000355, 36.39999999999999147, 2.499999999999996891 ) ) ;
#15843=EDGE_CURVE ( 'NONE', #13521, #14942, #1455, .T. ) ;
#15849=CARTESIAN_POINT ( 'NONE',  ( 10.00000000000000000, 18.79999999999999361, -2.500000000000003109 ) ) ;
#15852=EDGE_CURVE ( 'NONE', #12298, #14652, #14191, .T. ) ;
#15854=ORIENTED_EDGE ( 'NONE', *, *, #11573, .T. ) ;
#15863=TOROIDAL_SURFACE ( 'NONE', #7859, 9.000000000000003553, 0.9999999999999991118 ) ;
#15865=CARTESIAN_POINT ( 'NONE',  ( -1.734723475976807094E-15, 36.39999999999999147, -2.500000000000000000 ) ) ;
#15870=DIRECTION ( 'NONE',  ( -0.000000000000000000, -1.000000000000000000, -0.000000000000000000 ) ) ;
#15871=CARTESIAN_POINT ( 'NONE',  ( -1.734723475976807094E-15, 23.19999999999999574, -2.500000000000000000 ) ) ;
#15881=AXIS2_PLACEMENT_3D ( 'NONE', #5320, #13755, #15341 ) ;
#15884=EDGE_CURVE ( 'NONE', #3649, #8594, #12750, .T. ) ;
#15887=DIRECTION ( 'NONE',  ( -3.469446951953613696E-16, -0.000000000000000000, -1.000000000000000000 ) ) ;
#15888=CARTESIAN_POINT ( 'NONE',  ( 9.000000000000005329, 18.79999999999999361, 2.499999999999997335 ) ) ;
#15889=VERTEX_POINT ( 'NONE', #5523 ) ;
#15892=FACE_OUTER_BOUND ( 'NONE', #11791, .T. ) ;
#15896=TOROIDAL_SURFACE ( 'NONE', #2590, 9.000000000000001776, 0.9999999999999991118 ) ;
#15900=CARTESIAN_POINT ( 'NONE',  ( -1.734723475976807094E-15, 25.39999999999999503, -11.50000000000000178 ) ) ;
#15920=CIRCLE ( 'NONE', #1156, 8.000000000000001776 ) ;
#15922=DIRECTION ( 'NONE',  ( 1.000000000000000000, 0.000000000000000000, 0.000000000000000000 ) ) ;
#15928=ORIENTED_EDGE ( 'NONE', *, *, #9660, .T. ) ;
#15930=DIRECTION ( 'NONE',  ( -1.000000000000000000, 0.000000000000000000, 4.336808689942021680E-16 ) ) ;
#15946=CARTESIAN_POINT ( 'NONE',  ( 9.000000000000005329, 43.00000000000000000, 2.499999999999997335 ) ) ;
#15950=ORIENTED_EDGE ( 'NONE', *, *, #3325, .F. ) ;
#15956=ORIENTED_EDGE ( 'NONE', *, *, #3400, .T. ) ;
#15957=DIRECTION ( 'NONE',  ( -1.000000000000000000, 0.000000000000000000, 4.336808689942021680E-16 ) ) ;
#15964=CIRCLE ( 'NONE', #7349, 0.9999999999999991118 ) ;
#15972=VERTEX_POINT ( 'NONE', #11717 ) ;
#15978=CARTESIAN_POINT ( 'NONE',  ( 8.000000000000005329, 16.59999999999999787, 2.499999999999997780 ) ) ;
#15982=VECTOR ( 'NONE', #6110, 1000.000000000000000 ) ;
#15988=DIRECTION ( 'NONE',  ( -0.000000000000000000, -1.000000000000000000, -0.000000000000000000 ) ) ;
#15990=VERTEX_POINT ( 'NONE', #17222 ) ;
#15993=ORIENTED_EDGE ( 'NONE', *, *, #1293, .T. ) ;
#15998=CYLINDRICAL_SURFACE ( 'NONE', #1910, 0.9999999999999991118 ) ;
#15999=DIRECTION ( 'NONE',  ( 1.000000000000000000, 0.000000000000000000, 0.000000000000000000 ) ) ;
#16001=CARTESIAN_POINT ( 'NONE',  ( -1.734723475976807094E-15, 29.79999999999999716, -2.500000000000000000 ) ) ;
#16003=AXIS2_PLACEMENT_3D ( 'NONE', #981, #10978, #18052 ) ;
#16010=DIRECTION ( 'NONE',  ( -0.000000000000000000, -1.000000000000000000, -0.000000000000000000 ) ) ;
#16020=EDGE_CURVE ( 'NONE', #13486, #4985, #1491, .T. ) ;
#16027=EDGE_CURVE ( 'NONE', #17274, #5475, #7389, .T. ) ;
#16028=DIRECTION ( 'NONE',  ( -3.469446951953613696E-16, -0.000000000000000000, -1.000000000000000000 ) ) ;
#16032=AXIS2_PLACEMENT_3D ( 'NONE', #17415, #16010, #1926 ) ;
#16070=AXIS2_PLACEMENT_3D ( 'NONE', #107, #15870, #3167 ) ;
#16079=AXIS2_PLACEMENT_3D ( 'NONE', #4238, #1369, #14432 ) ;
#16081=STYLED_ITEM('',(#18396),#2004);
#16087=CYLINDRICAL_SURFACE ( 'NONE', #9993, 0.9999999999999991118 ) ;
#16088=ORIENTED_EDGE ( 'NONE', *, *, #13222, .F. ) ;
#16096=EDGE_CURVE ( 'NONE', #14197, #5921, #427, .T. ) ;
#16107=CIRCLE ( 'NONE', #100, 10.00000000000000178 ) ;
#16108=DIRECTION ( 'NONE',  ( 1.000000000000000000, 0.000000000000000000, -4.336808689942021680E-16 ) ) ;
#16112=CYLINDRICAL_SURFACE ( 'NONE', #6873, 0.9999999999999991118 ) ;
#16116=ORIENTED_EDGE ( 'NONE', *, *, #5520, .F. ) ;
#16129=DIRECTION ( 'NONE',  ( 0.000000000000000000, 0.000000000000000000, -1.000000000000000000 ) ) ;
#16138=LINE ( 'NONE', #15849, #1270 ) ;
#16143=ORIENTED_EDGE ( 'NONE', *, *, #14601, .F. ) ;
#16157=ORIENTED_EDGE ( 'NONE', *, *, #12726, .T. ) ;
#16159=DIRECTION ( 'NONE',  ( 0.000000000000000000, 0.000000000000000000, -1.000000000000000000 ) ) ;
#16167=DIRECTION ( 'NONE',  ( -1.000000000000000000, 0.000000000000000000, 4.336808689942021680E-16 ) ) ;
#16171=EDGE_LOOP ( 'NONE', ( #10661, #16711, #17678, #5442 ) ) ;
#16173=CARTESIAN_POINT ( 'NONE',  ( -10.00000000000000000, 25.39999999999999503, 2.499999999999998224 ) ) ;
#16185=ADVANCED_FACE ( 'NONE', ( #10699 ), #3563, .T. ) ;
#16187=EDGE_CURVE ( 'NONE', #3470, #13534, #10358, .T. ) ;
#16203=ORIENTED_EDGE ( 'NONE', *, *, #11573, .F. ) ;
#16215=VERTEX_POINT ( 'NONE', #9035 ) ;
#16220=ORIENTED_EDGE ( 'NONE', *, *, #17754, .T. ) ;
#16223=SURFACE_STYLE_USAGE ( .BOTH. , #10735 ) ;
#16230=CLOSED_SHELL ( 'NONE', ( #2861, #8722, #5852, #33, #957, #12086, #11518, #6377, #2865, #13156 ) ) ;
#16232=EDGE_CURVE ( 'NONE', #11085, #17274, #601, .T. ) ;
#16235=CIRCLE ( 'NONE', #231, 10.00000000000000178 ) ;
#16237=DIRECTION ( 'NONE',  ( 0.000000000000000000, 0.000000000000000000, -1.000000000000000000 ) ) ;
#16244=DIRECTION ( 'NONE',  ( -1.000000000000000000, 0.000000000000000000, 4.336808689942021680E-16 ) ) ;
#16247=AXIS2_PLACEMENT_3D ( 'NONE', #13187, #5866, #14402 ) ;
#16264=CARTESIAN_POINT ( 'NONE',  ( -1.734723475976807094E-15, 25.39999999999999503, -2.500000000000000000 ) ) ;
#16267=VERTEX_POINT ( 'NONE', #9127 ) ;
#16275=CIRCLE ( 'NONE', #17776, 0.9999999999999991118 ) ;
#16279=FACE_OUTER_BOUND ( 'NONE', #3050, .T. ) ;
#16281=AXIS2_PLACEMENT_3D ( 'NONE', #3189, #17108, #15530 ) ;
#16287=ORIENTED_EDGE ( 'NONE', *, *, #7189, .T. ) ;
#16288=CARTESIAN_POINT ( 'NONE',  ( -1.734723475976807094E-15, 29.79999999999999716, -2.500000000000000000 ) ) ;
#16293=DIRECTION ( 'NONE',  ( -3.469446951953613696E-16, -0.000000000000000000, -1.000000000000000000 ) ) ;
#16303=DIRECTION ( 'NONE',  ( 0.000000000000000000, 0.000000000000000000, 1.000000000000000000 ) ) ;
#16307=DIRECTION ( 'NONE',  ( 0.000000000000000000, 0.000000000000000000, -1.000000000000000000 ) ) ;
#16310=DIRECTION ( 'NONE',  ( -1.000000000000000000, 0.000000000000000000, 4.336808689942021680E-16 ) ) ;
#16312=AXIS2_PLACEMENT_3D ( 'NONE', #2999, #11604, #8724 ) ;
#16313=ORIENTED_EDGE ( 'NONE', *, *, #18026, .F. ) ;
#16320=ORIENTED_EDGE ( 'NONE', *, *, #2712, .F. ) ;
#16325=AXIS2_PLACEMENT_3D ( 'NONE', #12295, #644, #5255 ) ;
#16328=CARTESIAN_POINT ( 'NONE',  ( 10.00000000000000355, 25.39999999999999503, 2.499999999999996891 ) ) ;
#16348=AXIS2_PLACEMENT_3D ( 'NONE', #3018, #13958, #9780 ) ;
#16350=EDGE_CURVE ( 'NONE', #8594, #12622, #8876, .T. ) ;
#16360=ADVANCED_FACE ( 'NONE', ( #6707 ), #5034, .T. ) ;
#16368=EDGE_CURVE ( 'NONE', #6179, #4921, #10040, .T. ) ;
#16370=CARTESIAN_POINT ( 'NONE',  ( -1.734723475976807094E-15, 18.79999999999999361, -2.500000000000000000 ) ) ;
#16372=TOROIDAL_SURFACE ( 'NONE', #16079, 9.000000000000001776, 0.9999999999999991118 ) ;
#16373=VECTOR ( 'NONE', #11751, 1000.000000000000000 ) ;
#16381=CARTESIAN_POINT ( 'NONE',  ( 9.000000000000001776, 36.39999999999999147, -2.500000000000002665 ) ) ;
#16383=EDGE_LOOP ( 'NONE', ( #1010, #3059, #10935, #13184 ) ) ;
#16388=DIRECTION ( 'NONE',  ( -3.469446951953613696E-16, -0.000000000000000000, -1.000000000000000000 ) ) ;
#16395=CARTESIAN_POINT ( 'NONE',  ( 9.000000000000005329, 25.39999999999999503, 2.499999999999997335 ) ) ;
#16406=EDGE_LOOP ( 'NONE', ( #10622, #7113, #9455, #16530 ) ) ;
#16407=( GEOMETRIC_REPRESENTATION_CONTEXT ( 3 ) GLOBAL_UNCERTAINTY_ASSIGNED_CONTEXT ( ( #12482 ) ) GLOBAL_UNIT_ASSIGNED_CONTEXT ( ( #443, #7753, #9328 ) ) REPRESENTATION_CONTEXT ( 'NONE', 'WORKASPACE' ) );
#16409=DIRECTION ( 'NONE',  ( 0.000000000000000000, 0.000000000000000000, -1.000000000000000000 ) ) ;
#16427=EDGE_CURVE ( 'NONE', #12786, #9963, #12132, .T. ) ;
#16428=ORIENTED_EDGE ( 'NONE', *, *, #2419, .F. ) ;
#16430=CARTESIAN_POINT ( 'NONE',  ( -10.00000000000000178, 25.39999999999999503, -2.500000000000001776 ) ) ;
#16444=CARTESIAN_POINT ( 'NONE',  ( 10.00000000000000000, 36.39999999999999147, -2.500000000000003109 ) ) ;
#16445=DIRECTION ( 'NONE',  ( -3.469446951953613696E-16, -0.000000000000000000, -1.000000000000000000 ) ) ;
#16446=CARTESIAN_POINT ( 'NONE',  ( -9.000000000000001776, 43.00000000000000000, 2.499999999999998224 ) ) ;
#16449=CYLINDRICAL_SURFACE ( 'NONE', #7041, 0.9999999999999991118 ) ;
#16456=DIRECTION ( 'NONE',  ( 1.000000000000000000, 0.000000000000000000, 0.000000000000000000 ) ) ;
#16458=ADVANCED_FACE ( 'NONE', ( #9764 ), #9487, .T. ) ;
#16465=CIRCLE ( 'NONE', #10533, 8.000000000000001776 ) ;
#16468=CARTESIAN_POINT ( 'NONE',  ( -8.000000000000001776, 38.59999999999999432, 2.499999999999998224 ) ) ;
#16471=CIRCLE ( 'NONE', #9345, 0.9999999999999991118 ) ;
#16474=DIRECTION ( 'NONE',  ( 0.000000000000000000, 0.000000000000000000, -1.000000000000000000 ) ) ;
#16476=DIRECTION ( 'NONE',  ( 0.000000000000000000, 0.000000000000000000, -1.000000000000000000 ) ) ;
#16478=EDGE_CURVE ( 'NONE', #10466, #8695, #18323, .T. ) ;
#16482=EDGE_CURVE ( 'NONE', #11926, #5429, #11527, .T. ) ;
#16485=DIRECTION ( 'NONE',  ( 0.000000000000000000, 0.000000000000000000, -1.000000000000000000 ) ) ;
#16493=DIRECTION ( 'NONE',  ( 0.000000000000000000, 0.000000000000000000, -1.000000000000000000 ) ) ;
#16496=ORIENTED_EDGE ( 'NONE', *, *, #10577, .T. ) ;
#16498=CARTESIAN_POINT ( 'NONE',  ( -1.734723475976807094E-15, 18.79999999999999361, -2.500000000000000000 ) ) ;
#16499=SHAPE_REPRESENTATION_RELATIONSHIP ( 'NONE' , 'NONE' ,  #7684, #18244 ) ;
#16502=AXIS2_PLACEMENT_3D ( 'NONE', #15070, #8004, #14900 ) ;
#16508=DIRECTION ( 'NONE',  ( -4.915049848600951133E-16, 0.000000000000000000, -1.000000000000000000 ) ) ;
#16515=DIRECTION ( 'NONE',  ( 1.000000000000000000, 0.000000000000000000, 0.000000000000000000 ) ) ;
#16528=AXIS2_PLACEMENT_3D ( 'NONE', #16583, #13688, #16307 ) ;
#16530=ORIENTED_EDGE ( 'NONE', *, *, #16482, .T. ) ;
#16531=EDGE_CURVE ( 'NONE', #7975, #2685, #14822, .T. ) ;
#16538=CLOSED_SHELL ( 'NONE', ( #1675, #5477, #13952, #1473, #3992, #1157, #9435, #1050, #6084, #12544 ) ) ;
#16546=DIRECTION ( 'NONE',  ( 0.000000000000000000, 0.000000000000000000, 1.000000000000000000 ) ) ;
#16549=ORIENTED_EDGE ( 'NONE', *, *, #8011, .T. ) ;
#16555=DIRECTION ( 'NONE',  ( 3.469446951953612217E-16, -0.000000000000000000, 1.000000000000000000 ) ) ;
#16559=AXIS2_PLACEMENT_3D ( 'NONE', #10305, #15988, #14597 ) ;
#16575=AXIS2_PLACEMENT_3D ( 'NONE', #1450, #7081, #12747 ) ;
#16580=DIRECTION ( 'NONE',  ( 1.000000000000000000, 0.000000000000000000, 0.000000000000000000 ) ) ;
#16583=CARTESIAN_POINT ( 'NONE',  ( -1.734723475976807094E-15, 34.19999999999999574, -2.500000000000000000 ) ) ;
#16587=CARTESIAN_POINT ( 'NONE',  ( 8.000000000000005329, 40.79999999999999716, 2.499999999999997780 ) ) ;
#16592=ORIENTED_EDGE ( 'NONE', *, *, #16350, .T. ) ;
#16594=EDGE_CURVE ( 'NONE', #9655, #15102, #1800, .T. ) ;
#16597=UNCERTAINTY_MEASURE_WITH_UNIT (LENGTH_MEASURE( 1.000000000000000082E-05 ), #15648, 'distance_accuracy_value', 'NONE');
#16599=AXIS2_PLACEMENT_3D ( 'NONE', #18185, #5455, #12129 ) ;
#16616=DIRECTION ( 'NONE',  ( -3.469446951953613696E-16, -0.000000000000000000, -1.000000000000000000 ) ) ;
#16619=CARTESIAN_POINT ( 'NONE',  ( -10.00000000000000178, 27.59999999999999432, -2.500000000000001776 ) ) ;
#16637=CIRCLE ( 'NONE', #16325, 0.9999999999999991118 ) ;
#16640=ORIENTED_EDGE ( 'NONE', *, *, #14069, .F. ) ;
#16646=ORIENTED_EDGE ( 'NONE', *, *, #14092, .F. ) ;
#16651=FACE_OUTER_BOUND ( 'NONE', #4456, .T. ) ;
#16663=CYLINDRICAL_SURFACE ( 'NONE', #15049, 0.9999999999999991118 ) ;
#16671=FACE_OUTER_BOUND ( 'NONE', #3343, .T. ) ;
#16672=FACE_OUTER_BOUND ( 'NONE', #9233, .T. ) ;
#16679=CIRCLE ( 'NONE', #15498, 8.000000000000001776 ) ;
#16688=ORIENTED_EDGE ( 'NONE', *, *, #15392, .T. ) ;
#16695=EDGE_CURVE ( 'NONE', #3919, #12413, #13934, .T. ) ;
#16697=MECHANICAL_DESIGN_GEOMETRIC_PRESENTATION_REPRESENTATION('',(#2765),#8659);
#16701=CARTESIAN_POINT ( 'NONE',  ( -9.000000000000003553, 27.59999999999999432, -2.500000000000001776 ) ) ;
#16703=ORIENTED_EDGE ( 'NONE', *, *, #1845, .F. ) ;
#16704=CARTESIAN_POINT ( 'NONE',  ( 10.00000000000000355, 29.79999999999999716, 2.499999999999996891 ) ) ;
#16705=ORIENTED_EDGE ( 'NONE', *, *, #16368, .T. ) ;
#16711=ORIENTED_EDGE ( 'NONE', *, *, #6880, .F. ) ;
#16720=EDGE_CURVE ( 'NONE', #13359, #1006, #1799, .T. ) ;
#16722=EDGE_CURVE ( 'NONE', #15166, #17010, #13333, .T. ) ;
#16724=CIRCLE ( 'NONE', #3669, 0.9999999999999991118 ) ;
#16728=DIRECTION ( 'NONE',  ( -4.915049848600951133E-16, 0.000000000000000000, -1.000000000000000000 ) ) ;
#16731=DIRECTION ( 'NONE',  ( -1.000000000000000000, 0.000000000000000000, 4.336808689942021680E-16 ) ) ;
#16732=FACE_OUTER_BOUND ( 'NONE', #923, .T. ) ;
#16733=DIRECTION ( 'NONE',  ( -0.000000000000000000, -1.000000000000000000, -0.000000000000000000 ) ) ;
#16735=EDGE_LOOP ( 'NONE', ( #10121, #5963, #2959, #14412 ) ) ;
#16742=FACE_OUTER_BOUND ( 'NONE', #3313, .T. ) ;
#16745=AXIS2_PLACEMENT_3D ( 'NONE', #14923, #12380, #16485 ) ;
#16746=FACE_OUTER_BOUND ( 'NONE', #2828, .T. ) ;
#16748=CARTESIAN_POINT ( 'NONE',  ( 8.000000000000001776, 18.79999999999999361, -2.500000000000002220 ) ) ;
#16749=CARTESIAN_POINT ( 'NONE',  ( 0.000000000000000000, 36.39999999999999147, 2.500000000000000000 ) ) ;
#16756=FACE_OUTER_BOUND ( 'NONE', #59, .T. ) ;
#16764=EDGE_CURVE ( 'NONE', #4547, #14275, #10206, .T. ) ;
#16775=CARTESIAN_POINT ( 'NONE',  ( -8.000000000000003553, 18.79999999999999361, -2.500000000000001776 ) ) ;
#16777=UNCERTAINTY_MEASURE_WITH_UNIT (LENGTH_MEASURE( 1.000000000000000082E-05 ), #5096, 'distance_accuracy_value', 'NONE');
#16778=DIRECTION ( 'NONE',  ( -0.000000000000000000, -1.000000000000000000, -0.000000000000000000 ) ) ;
#16781=ORIENTED_EDGE ( 'NONE', *, *, #18063, .F. ) ;
#16784=AXIS2_PLACEMENT_3D ( 'NONE', #10222, #420, #14229 ) ;
#16791=VECTOR ( 'NONE', #8118, 1000.000000000000000 ) ;
#16794=ORIENTED_EDGE ( 'NONE', *, *, #13744, .T. ) ;
#16796=ORIENTED_EDGE ( 'NONE', *, *, #5062, .T. ) ;
#16797=CIRCLE ( 'NONE', #9944, 0.9999999999999991118 ) ;
#16801=ORIENTED_EDGE ( 'NONE', *, *, #17359, .F. ) ;
#16810=ORIENTED_EDGE ( 'NONE', *, *, #14316, .T. ) ;
#16815=DIRECTION ( 'NONE',  ( -1.000000000000000000, 0.000000000000000000, 4.336808689942021680E-16 ) ) ;
#16826=AXIS2_PLACEMENT_3D ( 'NONE', #18127, #16728, #4003 ) ;
#16832=EDGE_CURVE ( 'NONE', #6613, #17767, #14232, .T. ) ;
#16835=CYLINDRICAL_SURFACE ( 'NONE', #5505, 0.9999999999999991118 ) ;
#16836=ADVANCED_FACE ( 'NONE', ( #5026 ), #9190, .T. ) ;
#16839=FACE_OUTER_BOUND ( 'NONE', #13543, .T. ) ;
#16840=DIRECTION ( 'NONE',  ( -3.373073425510457965E-16, 0.000000000000000000, -1.000000000000000000 ) ) ;
#16845=DIRECTION ( 'NONE',  ( -1.000000000000000000, 0.000000000000000000, 4.336808689942021680E-16 ) ) ;
#16847=CIRCLE ( 'NONE', #10291, 10.00000000000000178 ) ;
#16849=AXIS2_PLACEMENT_3D ( 'NONE', #15888, #8917, #6046 ) ;
#16852=UNCERTAINTY_MEASURE_WITH_UNIT (LENGTH_MEASURE( 1.000000000000000082E-05 ), #3873, 'distance_accuracy_value', 'NONE');
#16867=CARTESIAN_POINT ( 'NONE',  ( -10.00000000000000178, 20.99999999999999289, -2.500000000000001776 ) ) ;
#16869=CARTESIAN_POINT ( 'NONE',  ( -1.734723475976807094E-15, 16.59999999999999787, -2.500000000000000000 ) ) ;
#16874=AXIS2_PLACEMENT_3D ( 'NONE', #2513, #8141, #13802 ) ;
#16878=( NAMED_UNIT ( * ) SI_UNIT ( $, .STERADIAN. ) SOLID_ANGLE_UNIT ( ) );
#16880=AXIS2_PLACEMENT_3D ( 'NONE', #12563, #6905, #18249 ) ;
#16884=EDGE_LOOP ( 'NONE', ( #10386, #8645, #16705, #9629 ) ) ;
#16885=CIRCLE ( 'NONE', #9464, 0.9999999999999991118 ) ;
#16887=( GEOMETRIC_REPRESENTATION_CONTEXT ( 3 ) GLOBAL_UNCERTAINTY_ASSIGNED_CONTEXT ( ( #8402 ) ) GLOBAL_UNIT_ASSIGNED_CONTEXT ( ( #15835, #14066, #1559 ) ) REPRESENTATION_CONTEXT ( 'NONE', 'WORKASPACE' ) );
#16914=CARTESIAN_POINT ( 'NONE',  ( -1.734723475976807094E-15, 27.59999999999999432, -2.500000000000000000 ) ) ;
#16916=ORIENTED_EDGE ( 'NONE', *, *, #12720, .T. ) ;
#16926=EDGE_CURVE ( 'NONE', #2439, #10092, #14217, .T. ) ;
#16927=CIRCLE ( 'NONE', #16032, 10.00000000000000000 ) ;
#16940=AXIS2_PLACEMENT_3D ( 'NONE', #9024, #13557, #6428 ) ;
#16942=ORIENTED_EDGE ( 'NONE', *, *, #16695, .F. ) ;
#16945=EDGE_CURVE ( 'NONE', #9963, #17338, #11884, .T. ) ;
#16952=ORIENTED_EDGE ( 'NONE', *, *, #8137, .T. ) ;
#16958=AXIS2_PLACEMENT_3D ( 'NONE', #4575, #7165, #15709 ) ;
#16960=UNCERTAINTY_MEASURE_WITH_UNIT (LENGTH_MEASURE( 1.000000000000000082E-05 ), #13427, 'distance_accuracy_value', 'NONE');
#16961=CIRCLE ( 'NONE', #6287, 0.9999999999999991118 ) ;
#16971=VECTOR ( 'NONE', #3427, 1000.000000000000000 ) ;
#16977=DIRECTION ( 'NONE',  ( 3.469446951953612217E-16, -0.000000000000000000, 1.000000000000000000 ) ) ;
#16988=TOROIDAL_SURFACE ( 'NONE', #15500, 9.000000000000001776, 0.9999999999999991118 ) ;
#16990=EDGE_LOOP ( 'NONE', ( #17743, #10666, #6004, #10258 ) ) ;
#16992=DIRECTION ( 'NONE',  ( 0.000000000000000000, 0.000000000000000000, -1.000000000000000000 ) ) ;
#16999=AXIS2_PLACEMENT_3D ( 'NONE', #8665, #7278, #347 ) ;
#17000=DIRECTION ( 'NONE',  ( 0.000000000000000000, 0.000000000000000000, -1.000000000000000000 ) ) ;
#17003=ORIENTED_EDGE ( 'NONE', *, *, #477, .F. ) ;
#17010=VERTEX_POINT ( 'NONE', #13830 ) ;
#17015=DIRECTION ( 'NONE',  ( -0.000000000000000000, -1.000000000000000000, -0.000000000000000000 ) ) ;
#17020=DIRECTION ( 'NONE',  ( -3.469446951953613696E-16, -0.000000000000000000, -1.000000000000000000 ) ) ;
#17032=EDGE_CURVE ( 'NONE', #8512, #15647, #8576, .T. ) ;
#17033=ORIENTED_EDGE ( 'NONE', *, *, #16478, .F. ) ;
#17037=CARTESIAN_POINT ( 'NONE',  ( -1.734723475976807094E-15, 27.59999999999999432, -2.500000000000000000 ) ) ;
#17046=DIRECTION ( 'NONE',  ( -3.469446951953613696E-16, -0.000000000000000000, -1.000000000000000000 ) ) ;
#17053=ADVANCED_FACE ( 'NONE', ( #5209 ), #6686, .T. ) ;
#17059=DIRECTION ( 'NONE',  ( 1.000000000000000000, 0.000000000000000000, 0.000000000000000000 ) ) ;
#17066=FACE_OUTER_BOUND ( 'NONE', #15561, .T. ) ;
#17089=DIRECTION ( 'NONE',  ( 0.000000000000000000, 0.000000000000000000, -1.000000000000000000 ) ) ;
#17091=FACE_OUTER_BOUND ( 'NONE', #3825, .T. ) ;
#17099=VECTOR ( 'NONE', #17763, 1000.000000000000000 ) ;
#17100=CARTESIAN_POINT ( 'NONE',  ( 8.000000000000001776, 23.19999999999999574, -2.500000000000002220 ) ) ;
#17108=DIRECTION ( 'NONE',  ( -3.469446951953613696E-16, -0.000000000000000000, -1.000000000000000000 ) ) ;
#17112=DIRECTION ( 'NONE',  ( 0.000000000000000000, 0.000000000000000000, -1.000000000000000000 ) ) ;
#17114=EDGE_CURVE ( 'NONE', #13741, #14997, #17811, .T. ) ;
#17119=CIRCLE ( 'NONE', #9106, 8.000000000000003553 ) ;
#17122=CARTESIAN_POINT ( 'NONE',  ( -1.734723475976807094E-15, 38.59999999999999432, -2.500000000000000000 ) ) ;
#17133=CIRCLE ( 'NONE', #9108, 0.9999999999999991118 ) ;
#17142=ORIENTED_EDGE ( 'NONE', *, *, #870, .F. ) ;
#17151=DIRECTION ( 'NONE',  ( 1.000000000000000000, 0.000000000000000000, -4.336808689942021680E-16 ) ) ;
#17157=ORIENTED_EDGE ( 'NONE', *, *, #11571, .F. ) ;
#17159=CARTESIAN_POINT ( 'NONE',  ( 9.000000000000000000, 36.39999999999999147, -2.500000000000001332 ) ) ;
#17171=CIRCLE ( 'NONE', #16575, 8.000000000000001776 ) ;
#17179=CIRCLE ( 'NONE', #276, 0.9999999999999991118 ) ;
#17183=ORIENTED_EDGE ( 'NONE', *, *, #17501, .T. ) ;
#17187=DIRECTION ( 'NONE',  ( -0.000000000000000000, -1.000000000000000000, -0.000000000000000000 ) ) ;
#17198=DIRECTION ( 'NONE',  ( -1.000000000000000000, 0.000000000000000000, 0.000000000000000000 ) ) ;
#17202=( GEOMETRIC_REPRESENTATION_CONTEXT ( 3 ) GLOBAL_UNCERTAINTY_ASSIGNED_CONTEXT ( ( #16597 ) ) GLOBAL_UNIT_ASSIGNED_CONTEXT ( ( #15648, #537, #4696 ) ) REPRESENTATION_CONTEXT ( 'NONE', 'WORKASPACE' ) );
#17222=CARTESIAN_POINT ( 'NONE',  ( 9.999999999999998224, 18.79999999999999361, -2.500000000000001776 ) ) ;
#17224=DIRECTION ( 'NONE',  ( 0.000000000000000000, 0.000000000000000000, -1.000000000000000000 ) ) ;
#17234=CARTESIAN_POINT ( 'NONE',  ( 0.000000000000000000, 34.19999999999999574, 2.500000000000000000 ) ) ;
#17249=ORIENTED_EDGE ( 'NONE', *, *, #17898, .F. ) ;
#17252=AXIS2_PLACEMENT_3D ( 'NONE', #12888, #8530, #1686 ) ;
#17253=CARTESIAN_POINT ( 'NONE',  ( -8.000000000000003553, 31.99999999999999289, -2.500000000000001776 ) ) ;
#17265=ORIENTED_EDGE ( 'NONE', *, *, #15775, .T. ) ;
#17274=VERTEX_POINT ( 'NONE', #9828 ) ;
#17277=DIRECTION ( 'NONE',  ( 0.000000000000000000, 0.000000000000000000, -1.000000000000000000 ) ) ;
#17280=AXIS2_PLACEMENT_3D ( 'NONE', #16869, #16778, #12484 ) ;
#17286=DIRECTION ( 'NONE',  ( -1.000000000000000000, 0.000000000000000000, 0.000000000000000000 ) ) ;
#17290=ADVANCED_FACE ( 'NONE', ( #2803 ), #3570, .T. ) ;
#17297=AXIS2_PLACEMENT_3D ( 'NONE', #4031, #6813, #16476 ) ;
#17306=EDGE_LOOP ( 'NONE', ( #16640, #11352, #14223, #16220 ) ) ;
#17315=VECTOR ( 'NONE', #11957, 1000.000000000000000 ) ;
#17326=TOROIDAL_SURFACE ( 'NONE', #17910, 9.000000000000003553, 0.9999999999999991118 ) ;
#17329=CARTESIAN_POINT ( 'NONE',  ( 9.000000000000001776, 16.59999999999999787, -2.500000000000002665 ) ) ;
#17331=LINE ( 'NONE', #4414, #2192 ) ;
#17334=ORIENTED_EDGE ( 'NONE', *, *, #2747, .F. ) ;
#17338=VERTEX_POINT ( 'NONE', #16587 ) ;
#17339=( GEOMETRIC_REPRESENTATION_CONTEXT ( 3 ) GLOBAL_UNCERTAINTY_ASSIGNED_CONTEXT ( ( #1372 ) ) GLOBAL_UNIT_ASSIGNED_CONTEXT ( ( #11257, #2838, #9952 ) ) REPRESENTATION_CONTEXT ( 'NONE', 'WORKASPACE' ) );
#17357=VERTEX_POINT ( 'NONE', #2495 ) ;
#17359=EDGE_CURVE ( 'NONE', #14942, #9017, #16637, .T. ) ;
#17362=DIRECTION ( 'NONE',  ( -1.000000000000000000, 0.000000000000000000, 4.336808689942021680E-16 ) ) ;
#17369=VERTEX_POINT ( 'NONE', #4892 ) ;
#17373=DIRECTION ( 'NONE',  ( 0.000000000000000000, 0.000000000000000000, 1.000000000000000000 ) ) ;
#17383=CIRCLE ( 'NONE', #474, 0.9999999999999991118 ) ;
#17396=ORIENTED_EDGE ( 'NONE', *, *, #7152, .F. ) ;
#17398=CIRCLE ( 'NONE', #15306, 8.000000000000003553 ) ;
#17415=CARTESIAN_POINT ( 'NONE',  ( -1.734723475976807094E-15, 38.59999999999999432, -2.500000000000000000 ) ) ;
#17420=DIRECTION ( 'NONE',  ( 3.469446951953612217E-16, -0.000000000000000000, 1.000000000000000000 ) ) ;
#17434=STYLED_ITEM('',(#18396),#14214);
#17436=VECTOR ( 'NONE', #9488, 1000.000000000000000 ) ;
#17453=AXIS2_PLACEMENT_3D ( 'NONE', #7064, #34, #11328 ) ;
#17456=DIRECTION ( 'NONE',  ( 0.000000000000000000, 0.000000000000000000, -1.000000000000000000 ) ) ;
#17461=PRODUCT_DEFINITION_SHAPE ( 'NONE', 'NONE',  #2334 ) ;
#17462=CARTESIAN_POINT ( 'NONE',  ( -1.734723475976807094E-15, 40.79999999999999716, -10.50000000000000178 ) ) ;
#17467=DIRECTION ( 'NONE',  ( -0.000000000000000000, -1.000000000000000000, -0.000000000000000000 ) ) ;
#17469=DIRECTION ( 'NONE',  ( 0.000000000000000000, 0.000000000000000000, -1.000000000000000000 ) ) ;
#17479=CIRCLE ( 'NONE', #10030, 10.00000000000000000 ) ;
#17486=FACE_OUTER_BOUND ( 'NONE', #9819, .T. ) ;
#17501=EDGE_CURVE ( 'NONE', #1278, #5475, #327, .T. ) ;
#17509=DIRECTION ( 'NONE',  ( 0.000000000000000000, 0.000000000000000000, -1.000000000000000000 ) ) ;
#17513=CARTESIAN_POINT ( 'NONE',  ( 9.000000000000005329, 27.59999999999999432, 2.499999999999997335 ) ) ;
#17522=FACE_OUTER_BOUND ( 'NONE', #832, .T. ) ;
#17528=EDGE_CURVE ( 'NONE', #5839, #9649, #820, .T. ) ;
#17529=ORIENTED_EDGE ( 'NONE', *, *, #1984, .F. ) ;
#17531=DIRECTION ( 'NONE',  ( -4.915049848600951133E-16, 0.000000000000000000, -1.000000000000000000 ) ) ;
#17534=CARTESIAN_POINT ( 'NONE',  ( -1.734723475976807094E-15, 27.59999999999999432, -2.500000000000000000 ) ) ;
#17540=ORIENTED_EDGE ( 'NONE', *, *, #11117, .T. ) ;
#17541=VERTEX_POINT ( 'NONE', #17809 ) ;
#17545=EDGE_CURVE ( 'NONE', #7045, #17369, #1518, .T. ) ;
#17548=ORIENTED_EDGE ( 'NONE', *, *, #1453, .F. ) ;
#17549=TOROIDAL_SURFACE ( 'NONE', #13657, 9.000000000000003553, 0.9999999999999991118 ) ;
#17552=ORIENTED_EDGE ( 'NONE', *, *, #4781, .T. ) ;
#17553=CARTESIAN_POINT ( 'NONE',  ( 0.000000000000000000, 38.59999999999999432, 2.500000000000000000 ) ) ;
#17563=ORIENTED_EDGE ( 'NONE', *, *, #13749, .F. ) ;
#17568=AXIS2_PLACEMENT_3D ( 'NONE', #6851, #12505, #2789 ) ;
#17569=ADVANCED_FACE ( 'NONE', ( #15011 ), #13347, .T. ) ;
#17571=STYLED_ITEM('',(#18396),#1553);
#17574=ADVANCED_FACE ( 'NONE', ( #6556 ), #10975, .T. ) ;
#17579=FACE_OUTER_BOUND ( 'NONE', #1867, .T. ) ;
#17580=TOROIDAL_SURFACE ( 'NONE', #5699, 9.000000000000001776, 0.9999999999999991118 ) ;
#17582=TOROIDAL_SURFACE ( 'NONE', #5984, 9.000000000000001776, 0.9999999999999991118 ) ;
#17589=FACE_OUTER_BOUND ( 'NONE', #3499, .T. ) ;
#17597=CIRCLE ( 'NONE', #17877, 8.000000000000003553 ) ;
#17603=CARTESIAN_POINT ( 'NONE',  ( -1.734723475976807094E-15, 38.59999999999999432, -11.50000000000000178 ) ) ;
#17606=ORIENTED_EDGE ( 'NONE', *, *, #16594, .F. ) ;
#17611=VERTEX_POINT ( 'NONE', #12569 ) ;
#17618=ORIENTED_EDGE ( 'NONE', *, *, #7508, .F. ) ;
#17624=DIRECTION ( 'NONE',  ( 1.000000000000000000, 0.000000000000000000, 0.000000000000000000 ) ) ;
#17628=FACE_OUTER_BOUND ( 'NONE', #11037, .T. ) ;
#17630=EDGE_CURVE ( 'NONE', #4921, #6179, #28, .T. ) ;
#17635=ORIENTED_EDGE ( 'NONE', *, *, #3276, .T. ) ;
#17638=CARTESIAN_POINT ( 'NONE',  ( -1.734723475976807094E-15, 38.59999999999999432, -12.50000000000000000 ) ) ;
#17639=DIRECTION ( 'NONE',  ( -4.915049848600951133E-16, 0.000000000000000000, -1.000000000000000000 ) ) ;
#17640=EDGE_CURVE ( 'NONE', #9378, #6645, #9198, .T. ) ;
#17648=DIRECTION ( 'NONE',  ( -0.000000000000000000, -1.000000000000000000, -0.000000000000000000 ) ) ;
#17657=CARTESIAN_POINT ( 'NONE',  ( -9.000000000000001776, 20.99999999999999289, 2.499999999999998224 ) ) ;
#17659=ORIENTED_EDGE ( 'NONE', *, *, #15525, .F. ) ;
#17669=CARTESIAN_POINT ( 'NONE',  ( -1.734723475976807094E-15, 36.39999999999999147, -2.500000000000000000 ) ) ;
#17672=VERTEX_POINT ( 'NONE', #3957 ) ;
#17675=EDGE_CURVE ( 'NONE', #6645, #9378, #1222, .T. ) ;
#17676=CYLINDRICAL_SURFACE ( 'NONE', #10106, 0.9999999999999991118 ) ;
#17678=ORIENTED_EDGE ( 'NONE', *, *, #5649, .T. ) ;
#17683=DIRECTION ( 'NONE',  ( 0.000000000000000000, 0.000000000000000000, -1.000000000000000000 ) ) ;
#17692=VERTEX_POINT ( 'NONE', #6996 ) ;
#17696=EDGE_CURVE ( 'NONE', #3919, #17357, #14545, .T. ) ;
#17706=AXIS2_PLACEMENT_3D ( 'NONE', #4932, #13546, #14877 ) ;
#17709=DIRECTION ( 'NONE',  ( -1.000000000000000000, 0.000000000000000000, 4.336808689942021680E-16 ) ) ;
#17712=DIRECTION ( 'NONE',  ( -1.000000000000000000, 0.000000000000000000, 4.336808689942021680E-16 ) ) ;
#17722=FACE_OUTER_BOUND ( 'NONE', #13905, .T. ) ;
#17729=VERTEX_POINT ( 'NONE', #18349 ) ;
#17736=CARTESIAN_POINT ( 'NONE',  ( 9.000000000000005329, 31.99999999999999289, 2.499999999999997335 ) ) ;
#17743=ORIENTED_EDGE ( 'NONE', *, *, #4226, .F. ) ;
#17750=FACE_OUTER_BOUND ( 'NONE', #6258, .T. ) ;
#17754=EDGE_CURVE ( 'NONE', #3449, #4719, #4765, .T. ) ;
#17757=ORIENTED_EDGE ( 'NONE', *, *, #10488, .T. ) ;
#17761=AXIS2_PLACEMENT_3D ( 'NONE', #14376, #7313, #290 ) ;
#17763=DIRECTION ( 'NONE',  ( 3.469446951953612217E-16, -0.000000000000000000, 1.000000000000000000 ) ) ;
#17766=VERTEX_POINT ( 'NONE', #338 ) ;
#17767=VERTEX_POINT ( 'NONE', #4775 ) ;
#17776=AXIS2_PLACEMENT_3D ( 'NONE', #3939, #10802, #18153 ) ;
#17777=AXIS2_PLACEMENT_3D ( 'NONE', #7845, #13498, #812 ) ;
#17779=CIRCLE ( 'NONE', #12702, 0.9999999999999991118 ) ;
#17782=CARTESIAN_POINT ( 'NONE',  ( 10.00000000000000355, 31.99999999999999289, 2.499999999999996891 ) ) ;
#17785=LINE ( 'NONE', #10700, #17436 ) ;
#17787=CARTESIAN_POINT ( 'NONE',  ( -10.00000000000000000, 23.19999999999999574, 2.499999999999996003 ) ) ;
#17798=AXIS2_PLACEMENT_3D ( 'NONE', #2377, #12179, #3572 ) ;
#17800=EDGE_LOOP ( 'NONE', ( #13800, #17757, #15014, #562 ) ) ;
#17801=CARTESIAN_POINT ( 'NONE',  ( -10.00000000000000000, 18.79999999999999361, 2.499999999999998224 ) ) ;
#17809=CARTESIAN_POINT ( 'NONE',  ( -8.000000000000003553, 34.19999999999999574, -2.500000000000001776 ) ) ;
#17811=CIRCLE ( 'NONE', #15133, 0.9999999999999991118 ) ;
#17813=ORIENTED_EDGE ( 'NONE', *, *, #3276, .F. ) ;
#17834=ORIENTED_EDGE ( 'NONE', *, *, #12935, .F. ) ;
#17848=ORIENTED_EDGE ( 'NONE', *, *, #1747, .F. ) ;
#17850=DIRECTION ( 'NONE',  ( 3.469446951953612217E-16, -0.000000000000000000, 1.000000000000000000 ) ) ;
#17853=TOROIDAL_SURFACE ( 'NONE', #16070, 9.000000000000003553, 0.9999999999999991118 ) ;
#17855=DIRECTION ( 'NONE',  ( 0.000000000000000000, 0.000000000000000000, -1.000000000000000000 ) ) ;
#17859=EDGE_CURVE ( 'NONE', #11611, #13188, #15440, .T. ) ;
#17862=DIRECTION ( 'NONE',  ( 0.000000000000000000, 0.000000000000000000, -1.000000000000000000 ) ) ;
#17875=FACE_OUTER_BOUND ( 'NONE', #12776, .T. ) ;
#17877=AXIS2_PLACEMENT_3D ( 'NONE', #3755, #8108, #13767 ) ;
#17885=LINE ( 'NONE', #5156, #16791 ) ;
#17898=EDGE_CURVE ( 'NONE', #1108, #3470, #16927, .T. ) ;
#17899=PRESENTATION_STYLE_ASSIGNMENT (( #16223 ) ) ;
#17903=EDGE_CURVE ( 'NONE', #17767, #17541, #145, .T. ) ;
#17910=AXIS2_PLACEMENT_3D ( 'NONE', #6211, #14760, #16237 ) ;
#17937=DIRECTION ( 'NONE',  ( -0.000000000000000000, -1.000000000000000000, -0.000000000000000000 ) ) ;
#17949=CARTESIAN_POINT ( 'NONE',  ( 8.000000000000000000, 43.00000000000000000, -2.500000000000000888 ) ) ;
#17954=CARTESIAN_POINT ( 'NONE',  ( -1.734723475976807094E-15, 20.99999999999999289, -2.500000000000000000 ) ) ;
#17958=DIRECTION ( 'NONE',  ( 0.000000000000000000, 0.000000000000000000, -1.000000000000000000 ) ) ;
#17966=CARTESIAN_POINT ( 'NONE',  ( -9.000000000000001776, 29.79999999999999716, 2.499999999999995559 ) ) ;
#17972=ORIENTED_EDGE ( 'NONE', *, *, #6834, .T. ) ;
#17976=ORIENTED_EDGE ( 'NONE', *, *, #15843, .F. ) ;
#17977=DIRECTION ( 'NONE',  ( 0.000000000000000000, 0.000000000000000000, 1.000000000000000000 ) ) ;
#18001=DIRECTION ( 'NONE',  ( -1.000000000000000000, 0.000000000000000000, 4.336808689942021680E-16 ) ) ;
#18002=( NAMED_UNIT ( * ) PLANE_ANGLE_UNIT ( ) SI_UNIT ( $, .RADIAN. ) );
#18004=CARTESIAN_POINT ( 'NONE',  ( 9.000000000000000000, 29.79999999999999716, -2.500000000000001332 ) ) ;
#18006=TOROIDAL_SURFACE ( 'NONE', #9966, 9.000000000000003553, 0.9999999999999991118 ) ;
#18008=CARTESIAN_POINT ( 'NONE',  ( -8.000000000000003553, 29.79999999999999716, -2.500000000000001776 ) ) ;
#18011=CARTESIAN_POINT ( 'NONE',  ( -9.000000000000001776, 18.79999999999999361, 2.499999999999995559 ) ) ;
#18012=EDGE_LOOP ( 'NONE', ( #5665, #8488, #13673, #15854 ) ) ;
#18021=ORIENTED_EDGE ( 'NONE', *, *, #11576, .T. ) ;
#18026=EDGE_CURVE ( 'NONE', #13741, #12298, #6250, .T. ) ;
#18029=MECHANICAL_DESIGN_GEOMETRIC_PRESENTATION_REPRESENTATION('',(#9693),#1731);
#18030=DIRECTION ( 'NONE',  ( 1.000000000000000000, 0.000000000000000000, -4.336808689942021680E-16 ) ) ;
#18033=CIRCLE ( 'NONE', #13266, 0.9999999999999991118 ) ;
#18034=ORIENTED_EDGE ( 'NONE', *, *, #13676, .T. ) ;
#18037=DIRECTION ( 'NONE',  ( 3.469446951953612217E-16, -0.000000000000000000, 1.000000000000000000 ) ) ;
#18045=DIRECTION ( 'NONE',  ( 1.000000000000000000, 0.000000000000000000, 0.000000000000000000 ) ) ;
#18046=AXIS2_PLACEMENT_3D ( 'NONE', #17966, #12458, #9590 ) ;
#18047=AXIS2_PLACEMENT_3D ( 'NONE', #5488, #6515, #13742 ) ;
#18050=CARTESIAN_POINT ( 'NONE',  ( 9.000000000000000000, 23.19999999999999574, -2.500000000000001332 ) ) ;
#18052=DIRECTION ( 'NONE',  ( 0.000000000000000000, 0.000000000000000000, -1.000000000000000000 ) ) ;
#18053=CIRCLE ( 'NONE', #13587, 10.00000000000000000 ) ;
#18057=CARTESIAN_POINT ( 'NONE',  ( 10.00000000000000355, 20.99999999999999289, 2.499999999999996891 ) ) ;
#18058=AXIS2_PLACEMENT_3D ( 'NONE', #16395, #17531, #17709 ) ;
#18060=CARTESIAN_POINT ( 'NONE',  ( -9.000000000000001776, 25.39999999999999503, 2.499999999999998224 ) ) ;
#18063=EDGE_CURVE ( 'NONE', #1200, #3107, #10401, .T. ) ;
#18069=DIRECTION ( 'NONE',  ( -4.915049848600951133E-16, 0.000000000000000000, -1.000000000000000000 ) ) ;
#18074=DIRECTION ( 'NONE',  ( -0.000000000000000000, -1.000000000000000000, -0.000000000000000000 ) ) ;
#18083=EDGE_CURVE ( 'NONE', #17611, #2412, #2014, .T. ) ;
#18086=UNCERTAINTY_MEASURE_WITH_UNIT (LENGTH_MEASURE( 1.000000000000000082E-05 ), #109, 'distance_accuracy_value', 'NONE');
#18089=ADVANCED_FACE ( 'NONE', ( #6532 ), #2432, .T. ) ;
#18099=MECHANICAL_DESIGN_GEOMETRIC_PRESENTATION_REPRESENTATION('',(#5411),#17339);
#18101=DIRECTION ( 'NONE',  ( 1.000000000000000000, 0.000000000000000000, 0.000000000000000000 ) ) ;
#18102=STYLED_ITEM('',(#18396),#7707);
#18104=DIRECTION ( 'NONE',  ( 0.000000000000000000, 0.000000000000000000, 1.000000000000000000 ) ) ;
#18105=ORIENTED_EDGE ( 'NONE', *, *, #314, .T. ) ;
#18116=UNCERTAINTY_MEASURE_WITH_UNIT (LENGTH_MEASURE( 1.000000000000000082E-05 ), #6927, 'distance_accuracy_value', 'NONE');
#18127=CARTESIAN_POINT ( 'NONE',  ( 9.000000000000005329, 20.99999999999999289, 2.499999999999997335 ) ) ;
#18141=FACE_OUTER_BOUND ( 'NONE', #15103, .T. ) ;
#18142=ADVANCED_FACE ( 'NONE', ( #11999 ), #17549, .T. ) ;
#18146=DIRECTION ( 'NONE',  ( -1.000000000000000000, 0.000000000000000000, 4.336808689942021680E-16 ) ) ;
#18148=DIRECTION ( 'NONE',  ( -0.000000000000000000, -1.000000000000000000, -0.000000000000000000 ) ) ;
#18153=DIRECTION ( 'NONE',  ( 0.000000000000000000, 0.000000000000000000, 1.000000000000000000 ) ) ;
#18169=CARTESIAN_POINT ( 'NONE',  ( -1.734723475976807094E-15, 31.99999999999999289, -2.500000000000000000 ) ) ;
#18170=VECTOR ( 'NONE', #13451, 1000.000000000000000 ) ;
#18174=ORIENTED_EDGE ( 'NONE', *, *, #7259, .F. ) ;
#18185=CARTESIAN_POINT ( 'NONE',  ( 0.000000000000000000, 43.00000000000000000, 2.500000000000000000 ) ) ;
#18186=TOROIDAL_SURFACE ( 'NONE', #4835, 9.000000000000001776, 0.9999999999999991118 ) ;
#18190=CARTESIAN_POINT ( 'NONE',  ( -9.000000000000003553, 18.79999999999999361, -2.500000000000001776 ) ) ;
#18195=DIRECTION ( 'NONE',  ( -1.000000000000000000, 0.000000000000000000, 4.336808689942021680E-16 ) ) ;
#18199=FACE_OUTER_BOUND ( 'NONE', #3359, .T. ) ;
#18202=VERTEX_POINT ( 'NONE', #14592 ) ;
#18213=DIRECTION ( 'NONE',  ( 0.000000000000000000, 0.000000000000000000, 1.000000000000000000 ) ) ;
#18218=ORIENTED_EDGE ( 'NONE', *, *, #15742, .T. ) ;
#18220=FACE_OUTER_BOUND ( 'NONE', #12889, .T. ) ;
#18229=CARTESIAN_POINT ( 'NONE',  ( -1.734723475976807094E-15, 27.59999999999999432, -2.500000000000000000 ) ) ;
#18236=EDGE_CURVE ( 'NONE', #1028, #1579, #4471, .T. ) ;
#18241=DIRECTION ( 'NONE',  ( 1.000000000000000000, 0.000000000000000000, 0.000000000000000000 ) ) ;
#18244=ADVANCED_BREP_SHAPE_REPRESENTATION ( '', ( #7672, #7822, #7707, #13807, #2004, #1553, #14621, #8199, #13775, #8351, #14214, #14659, #2247, #16940 ), #11010 ) ;
#18249=DIRECTION ( 'NONE',  ( -1.000000000000000000, 0.000000000000000000, 4.336808689942021680E-16 ) ) ;
#18251=DIRECTION ( 'NONE',  ( 3.469446951953612217E-16, -0.000000000000000000, 1.000000000000000000 ) ) ;
#18253=EDGE_CURVE ( 'NONE', #6645, #4921, #10400, .T. ) ;
#18254=CARTESIAN_POINT ( 'NONE',  ( -8.000000000000001776, 23.19999999999999574, 2.499999999999998224 ) ) ;
#18257=DIRECTION ( 'NONE',  ( -1.000000000000000000, 0.000000000000000000, 4.336808689942021680E-16 ) ) ;
#18261=DIRECTION ( 'NONE',  ( -0.000000000000000000, -1.000000000000000000, -0.000000000000000000 ) ) ;
#18266=VERTEX_POINT ( 'NONE', #11693 ) ;
#18278=TOROIDAL_SURFACE ( 'NONE', #1088, 9.000000000000001776, 0.9999999999999991118 ) ;
#18293=EDGE_CURVE ( 'NONE', #7975, #723, #11785, .T. ) ;
#18304=ORIENTED_EDGE ( 'NONE', *, *, #3829, .T. ) ;
#18318=CYLINDRICAL_SURFACE ( 'NONE', #15881, 0.9999999999999991118 ) ;
#18320=AXIS2_PLACEMENT_3D ( 'NONE', #9983, #3138, #7205 ) ;
#18321=AXIS2_PLACEMENT_3D ( 'NONE', #3745, #982, #10884 ) ;
#18323=LINE ( 'NONE', #16748, #5325 ) ;
#18330=EDGE_CURVE ( 'NONE', #5909, #904, #591, .T. ) ;
#18336=AXIS2_PLACEMENT_3D ( 'NONE', #13927, #15589, #18030 ) ;
#18340=CARTESIAN_POINT ( 'NONE',  ( 0.000000000000000000, 27.59999999999999432, 2.500000000000000000 ) ) ;
#18342=AXIS2_PLACEMENT_3D ( 'NONE', #3753, #15357, #16845 ) ;
#18344=FACE_OUTER_BOUND ( 'NONE', #10674, .T. ) ;
#18345=AXIS2_PLACEMENT_3D ( 'NONE', #11022, #16616, #18195 ) ;
#18349=CARTESIAN_POINT ( 'NONE',  ( -8.000000000000003553, 36.39999999999999147, -2.500000000000001776 ) ) ;
#18354=EDGE_CURVE ( 'NONE', #13234, #12374, #3897, .T. ) ;
#18360=CIRCLE ( 'NONE', #6183, 10.00000000000000178 ) ;
#18362=AXIS2_PLACEMENT_3D ( 'NONE', #10927, #10745, #11014 ) ;
#18364=EDGE_LOOP ( 'NONE', ( #13774, #14957, #16592, #13530 ) ) ;
#18368=CARTESIAN_POINT ( 'NONE',  ( -9.000000000000003553, 16.59999999999999787, -2.500000000000001776 ) ) ;
#18390=COLOUR_RGB('Light Blue',0.38,0.62,0.78);
#18391=FILL_AREA_STYLE_COLOUR('',#18390);
#18392=FILL_AREA_STYLE('',(#18391));
#18393=SURFACE_STYLE_FILL_AREA(#18392);
#18394=SURFACE_SIDE_STYLE('',(#18393));
#18395=SURFACE_STYLE_USAGE(.BOTH.,#18394);
#18396=PRESENTATION_STYLE_ASSIGNMENT((#18395));
ENDSEC;
END-ISO-10303-21;
